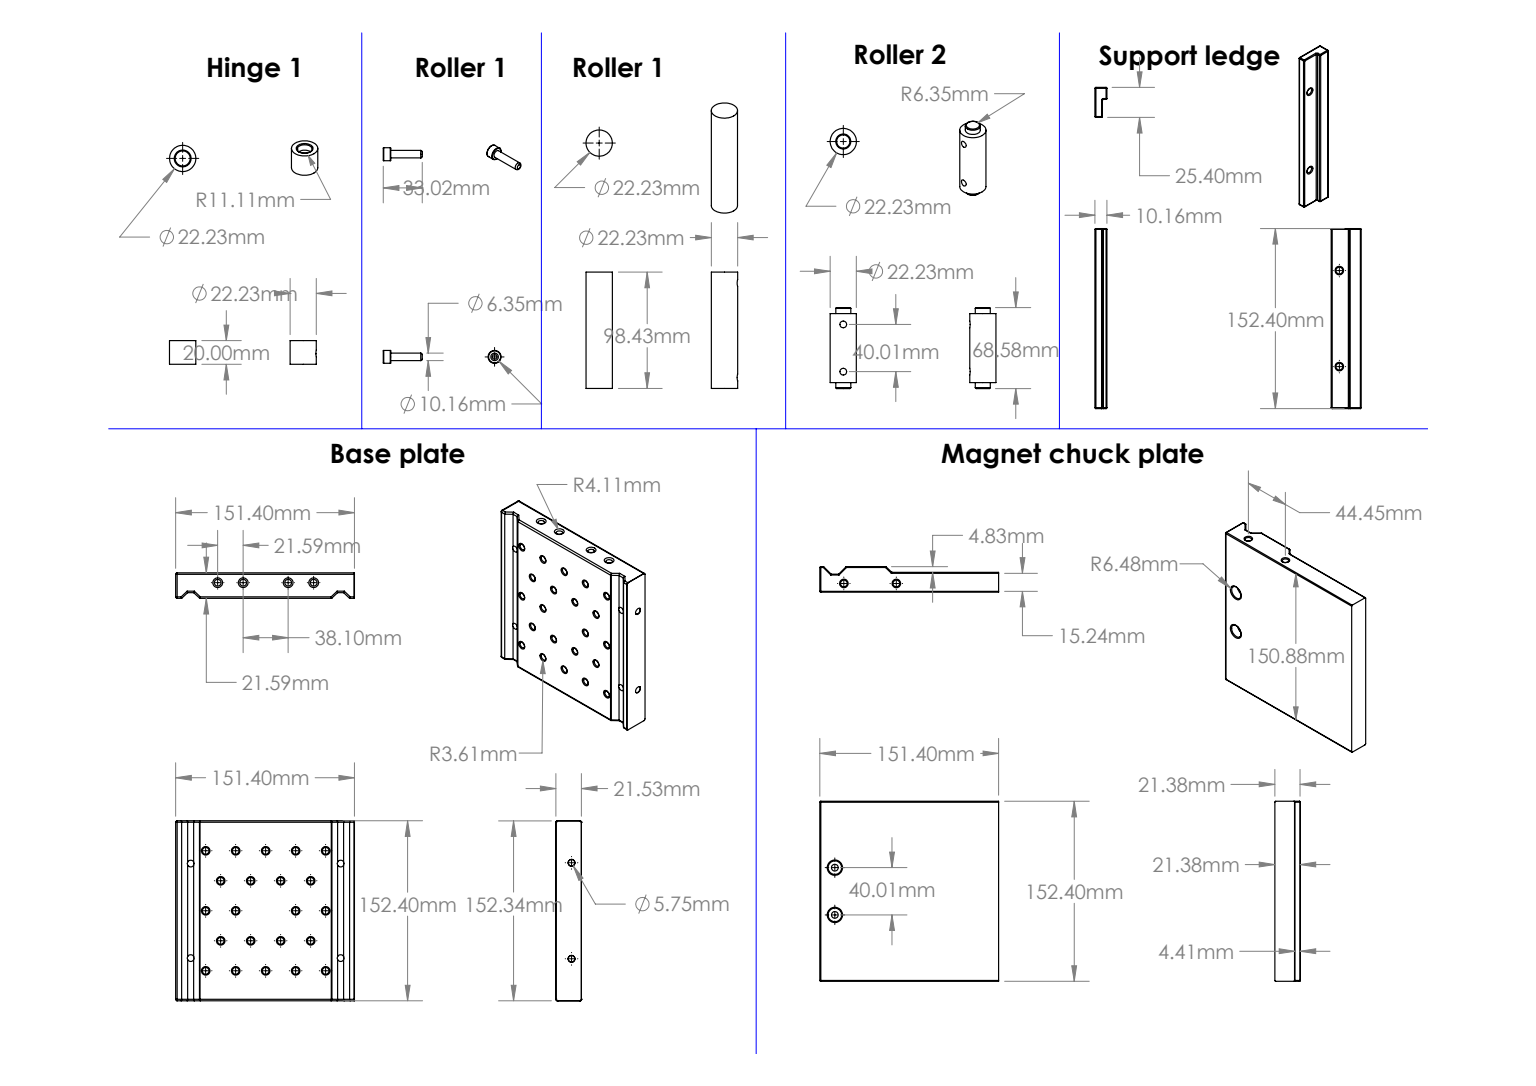
ISO-10303-21;
HEADER;
FILE_DESCRIPTION (('STEP AP214'),
    '1' );
FILE_NAME ('Magnet Chuck Plate.step',
    '2026-10-26T17:37:43',
    ( '' ),
    ( '' ),
    'SwSTEP 2.0',
    'SolidWorks 2024',
    '' );
FILE_SCHEMA (( 'AUTOMOTIVE_DESIGN' ));
ENDSEC;

DATA;
#1=EDGE_CURVE ( 'NONE', #5531, #18286, #22565, .T. ) ;
#10=CARTESIAN_POINT ( 'NONE',  ( 0.7620000000000000107, -3544.061999999999898, 2275.763800000000174 ) ) ;
#53=LINE ( 'NONE', #7432, #17005 ) ;
#82=LINE ( 'NONE', #12499, #17173 ) ;
#90=DIRECTION ( 'NONE',  ( 1.000000000000000000, 0.000000000000000000, 0.000000000000000000 ) ) ;
#100=ORIENTED_EDGE ( 'NONE', *, *, #20293, .T. ) ;
#116=ADVANCED_FACE ( 'NONE', ( #12202 ), #6711, .T. ) ;
#142=DIRECTION ( 'NONE',  ( 0.000000000000000000, 0.000000000000000000, 1.000000000000000000 ) ) ;
#171=DIRECTION ( 'NONE',  ( 0.000000000000000000, 1.000000000000000000, 0.000000000000000000 ) ) ;
#180=AXIS2_PLACEMENT_3D ( 'NONE', #4106, #4219, #18284 ) ;
#191=CARTESIAN_POINT ( 'NONE',  ( 20.32000000000000028, -3568.700000000000273, 2289.213099999999940 ) ) ;
#194=AXIS2_PLACEMENT_3D ( 'NONE', #19267, #12347, #20783 ) ;
#208=CARTESIAN_POINT ( 'NONE',  ( 64.76999999999999602, -3544.061999999999898, 2285.606299999999919 ) ) ;
#211=EDGE_CURVE ( 'NONE', #9937, #6734, #5182, .T. ) ;
#225=ORIENTED_EDGE ( 'NONE', *, *, #4542, .T. ) ;
#244=CIRCLE ( 'NONE', #16685, 5.714999999998999769 ) ;
#250=VECTOR ( 'NONE', #21152, 1000.000000000000000 ) ;
#253=CARTESIAN_POINT ( 'NONE',  ( 64.76999999999999602, -3543.299999999999727, 2289.213099999999940 ) ) ;
#254=ADVANCED_FACE ( 'NONE', ( #12432 ), #16297, .F. ) ;
#255=ADVANCED_FACE ( 'NONE', ( #18168 ), #10909, .F. ) ;
#259=DIRECTION ( 'NONE',  ( 0.000000000000000000, -1.000000000000000000, 0.000000000000000000 ) ) ;
#295=DIRECTION ( 'NONE',  ( -9.561467977825806485E-14, 1.000000000000000000, 0.000000000000000000 ) ) ;
#330=CIRCLE ( 'NONE', #16415, 0.7619999999999294005 ) ;
#355=ADVANCED_FACE ( 'NONE', ( #3996 ), #10792, .T. ) ;
#358=DIRECTION ( 'NONE',  ( 0.000000000000000000, 0.000000000000000000, 1.000000000000000000 ) ) ;
#363=AXIS2_PLACEMENT_3D ( 'NONE', #2504, #11180, #9647 ) ;
#389=AXIS2_PLACEMENT_3D ( 'NONE', #3368, #21197, #5143 ) ;
#392=ORIENTED_EDGE ( 'NONE', *, *, #12214, .T. ) ;
#400=CARTESIAN_POINT ( 'NONE',  ( 19.17699999999999960, -3639.502500000000055, 2295.829799999999977 ) ) ;
#403=DIRECTION ( 'NONE',  ( 1.000000000000000000, 0.000000000000000000, 0.000000000000000000 ) ) ;
#414=CIRCLE ( 'NONE', #13497, 3.606800000000021100 ) ;
#415=LINE ( 'NONE', #12612, #10639 ) ;
#438=VECTOR ( 'NONE', #18888, 1000.000000000000000 ) ;
#440=DIRECTION ( 'NONE',  ( 1.000000000000000000, 0.000000000000000000, 0.000000000000000000 ) ) ;
#441=CARTESIAN_POINT ( 'NONE',  ( 55.57575231171000496, -3544.061999999999898, 2275.763800000000174 ) ) ;
#460=TOROIDAL_SURFACE ( 'NONE', #16565, 6.476999999999000224, 0.7620000000000000107 ) ;
#476=AXIS2_PLACEMENT_3D ( 'NONE', #15163, #22181, #14935 ) ;
#492=CARTESIAN_POINT ( 'NONE',  ( 22.54063073453000143, -3695.699999999999818, 2275.763800000000174 ) ) ;
#504=AXIS2_PLACEMENT_3D ( 'NONE', #7643, #14804, #7882 ) ;
#508=ORIENTED_EDGE ( 'NONE', *, *, #16803, .F. ) ;
#510=CARTESIAN_POINT ( 'NONE',  ( 61.26424768829000556, -3695.699999999999818, 2280.589800000000196 ) ) ;
#520=LINE ( 'NONE', #7549, #8680 ) ;
#522=DIRECTION ( 'NONE',  ( 0.000000000000000000, 0.000000000000000000, 1.000000000000000000 ) ) ;
#555=ORIENTED_EDGE ( 'NONE', *, *, #7128, .T. ) ;
#580=DIRECTION ( 'NONE',  ( 0.000000000000000000, 0.000000000000000000, 1.000000000000000000 ) ) ;
#599=DIRECTION ( 'NONE',  ( 0.000000000000000000, 0.000000000000000000, 1.000000000000000000 ) ) ;
#602=ORIENTED_EDGE ( 'NONE', *, *, #20236, .T. ) ;
#616=ORIENTED_EDGE ( 'NONE', *, *, #16446, .F. ) ;
#626=AXIS2_PLACEMENT_3D ( 'NONE', #6837, #15624, #3186 ) ;
#629=DIRECTION ( 'NONE',  ( -1.000000000000000000, 0.000000000000000000, 0.000000000000000000 ) ) ;
#636=DIRECTION ( 'NONE',  ( 0.000000000000000000, -1.000000000000000000, 0.000000000000000000 ) ) ;
#649=AXIS2_PLACEMENT_3D ( 'NONE', #3890, #6955, #18185 ) ;
#651=ORIENTED_EDGE ( 'NONE', *, *, #14900, .F. ) ;
#654=DIRECTION ( 'NONE',  ( 0.000000000000000000, -1.000000000000000000, 0.000000000000000000 ) ) ;
#661=ADVANCED_FACE ( 'NONE', ( #9884 ), #22307, .T. ) ;
#665=AXIS2_PLACEMENT_3D ( 'NONE', #11297, #7552, #21854 ) ;
#701=ORIENTED_EDGE ( 'NONE', *, *, #13282, .T. ) ;
#725=LINE ( 'NONE', #14924, #438 ) ;
#743=DIRECTION ( 'NONE',  ( 0.000000000000000000, 0.000000000000000000, 1.000000000000000000 ) ) ;
#753=DIRECTION ( 'NONE',  ( -0.7071067811865975328, 0.000000000000000000, 0.7071067811864976127 ) ) ;
#762=EDGE_CURVE ( 'NONE', #1396, #13309, #12722, .T. ) ;
#789=CARTESIAN_POINT ( 'NONE',  ( 22.54063073453000143, -3543.299999999999727, 2275.763800000000174 ) ) ;
#821=DIRECTION ( 'NONE',  ( 0.000000000000000000, 0.000000000000000000, 1.000000000000000000 ) ) ;
#833=VERTEX_POINT ( 'NONE', #22769 ) ;
#834=ORIENTED_EDGE ( 'NONE', *, *, #2199, .T. ) ;
#841=FACE_OUTER_BOUND ( 'NONE', #17125, .T. ) ;
#851=ADVANCED_FACE ( 'NONE', ( #4969 ), #12116, .T. ) ;
#852=AXIS2_PLACEMENT_3D ( 'NONE', #21590, #20065, #5891 ) ;
#864=AXIS2_PLACEMENT_3D ( 'NONE', #15935, #8563, #21219 ) ;
#877=EDGE_LOOP ( 'NONE', ( #14414, #4341, #3151, #7613 ) ) ;
#880=DIRECTION ( 'NONE',  ( 1.000000000000000000, -0.000000000000000000, 1.224646799147353207E-16 ) ) ;
#885=ORIENTED_EDGE ( 'NONE', *, *, #19026, .T. ) ;
#915=DIRECTION ( 'NONE',  ( 1.000000000000000000, 0.000000000000000000, 0.000000000000000000 ) ) ;
#927=VECTOR ( 'NONE', #17929, 1000.000000000000000 ) ;
#942=ADVANCED_FACE ( 'NONE', ( #18087 ), #11055, .F. ) ;
#944=EDGE_CURVE ( 'NONE', #12459, #5100, #7542, .T. ) ;
#948=DIRECTION ( 'NONE',  ( 1.000000000000000000, 0.000000000000000000, 0.000000000000000000 ) ) ;
#993=LINE ( 'NONE', #6058, #8747 ) ;
#1013=DIRECTION ( 'NONE',  ( 0.000000000000000000, 0.000000000000000000, -1.000000000000000000 ) ) ;
#1036=ORIENTED_EDGE ( 'NONE', *, *, #20193, .F. ) ;
#1047=EDGE_LOOP ( 'NONE', ( #19998, #10354 ) ) ;
#1048=AXIS2_PLACEMENT_3D ( 'NONE', #4123, #18073, #7418 ) ;
#1052=EDGE_CURVE ( 'NONE', #8155, #9937, #725, .T. ) ;
#1069=ORIENTED_EDGE ( 'NONE', *, *, #7661, .F. ) ;
#1071=FACE_OUTER_BOUND ( 'NONE', #18282, .T. ) ;
#1081=AXIS2_PLACEMENT_3D ( 'NONE', #4745, #21035, #19158 ) ;
#1088=CARTESIAN_POINT ( 'NONE',  ( 2.859369265564648099, -3695.699999999999818, 2275.763800000091578 ) ) ;
#1109=AXIS2_PLACEMENT_3D ( 'NONE', #7606, #2336, #580 ) ;
#1134=VECTOR ( 'NONE', #15380, 1000.000000000000000 ) ;
#1151=DIRECTION ( 'NONE',  ( -0.6887494619146010688, 0.000000000000000000, 0.7249994335945012525 ) ) ;
#1177=CARTESIAN_POINT ( 'NONE',  ( 12.69999999999999929, -3599.497499999999945, 2288.971800000000258 ) ) ;
#1200=VERTEX_POINT ( 'NONE', #8469 ) ;
#1205=VERTEX_POINT ( 'NONE', #3299 ) ;
#1219=CARTESIAN_POINT ( 'NONE',  ( 64.76999999999999602, -3670.300000000000182, 2286.368300000000090 ) ) ;
#1222=ORIENTED_EDGE ( 'NONE', *, *, #2628, .T. ) ;
#1255=APPLICATION_CONTEXT ( 'configuration controlled 3d designs of mechanical parts and assemblies' ) ;
#1261=ADVANCED_FACE ( 'NONE', ( #17474 ), #5308, .T. ) ;
#1281=DIRECTION ( 'NONE',  ( 0.000000000000000000, 1.000000000000000000, 0.000000000000000000 ) ) ;
#1300=FACE_OUTER_BOUND ( 'NONE', #22874, .T. ) ;
#1301=VECTOR ( 'NONE', #7650, 1000.000000000000000 ) ;
#1306=DIRECTION ( 'NONE',  ( 0.000000000000000000, 0.000000000000000000, 1.000000000000000000 ) ) ;
#1321=CARTESIAN_POINT ( 'NONE',  ( 22.00181536726000076, -3694.938000000000102, 2275.224984633000076 ) ) ;
#1325=ADVANCED_FACE ( 'NONE', ( #21119 ), #14206, .F. ) ;
#1327=ORIENTED_EDGE ( 'NONE', *, *, #3052, .T. ) ;
#1343=EDGE_LOOP ( 'NONE', ( #9952, #15116, #508, #11219 ) ) ;
#1358=VECTOR ( 'NONE', #19375, 1000.000000000000000 ) ;
#1371=VERTEX_POINT ( 'NONE', #21695 ) ;
#1372=CIRCLE ( 'NONE', #12234, 5.714999999999999858 ) ;
#1396=VERTEX_POINT ( 'NONE', #17830 ) ;
#1409=CARTESIAN_POINT ( 'NONE',  ( 12.69999999999999929, -3599.497499999999945, 2296.591799999999694 ) ) ;
#1411=AXIS2_PLACEMENT_3D ( 'NONE', #10840, #17987, #14487 ) ;
#1414=VERTEX_POINT ( 'NONE', #7284 ) ;
#1421=SHAPE_REPRESENTATION ( 'Magnet Chuck Plate', ( #5611 ), #15735 ) ;
#1423=DIRECTION ( 'NONE',  ( 1.000000000000000000, 0.000000000000000000, 0.000000000000000000 ) ) ;
#1426=CARTESIAN_POINT ( 'NONE',  ( 61.26424768829000556, -3544.061999999999898, 2279.065800000000309 ) ) ;
#1428=DIRECTION ( 'NONE',  ( 0.000000000000000000, 0.000000000000000000, 1.000000000000000000 ) ) ;
#1439=CIRCLE ( 'NONE', #4438, 0.7619999999999294005 ) ;
#1444=CARTESIAN_POINT ( 'NONE',  ( 55.57575231171000496, -3544.061999999999898, 2275.001800000000003 ) ) ;
#1482=CARTESIAN_POINT ( 'NONE',  ( 6.985000000000999520, -3599.497499999999945, 2288.971800000000258 ) ) ;
#1484=VERTEX_POINT ( 'NONE', #13128 ) ;
#1496=ORIENTED_EDGE ( 'NONE', *, *, #16738, .F. ) ;
#1502=CARTESIAN_POINT ( 'NONE',  ( 20.32000000000000028, -3670.300000000000182, 2286.368300000000090 ) ) ;
#1509=EDGE_CURVE ( 'NONE', #7148, #4633, #7924, .T. ) ;
#1513=DIRECTION ( 'NONE',  ( 0.000000000000000000, 0.000000000000000000, 1.000000000000000000 ) ) ;
#1519=DIRECTION ( 'NONE',  ( -0.7071067811860285435, 0.000000000000000000, -0.7071067811870666020 ) ) ;
#1533=ORIENTED_EDGE ( 'NONE', *, *, #7543, .T. ) ;
#1537=ORIENTED_EDGE ( 'NONE', *, *, #16396, .F. ) ;
#1551=CARTESIAN_POINT ( 'NONE',  ( 151.6380000000000052, -3544.061999999999898, 2279.827800000000025 ) ) ;
#1558=EDGE_LOOP ( 'NONE', ( #1774, #9639 ) ) ;
#1571=ORIENTED_EDGE ( 'NONE', *, *, #2628, .F. ) ;
#1574=CARTESIAN_POINT ( 'NONE',  ( 11.65131536725999872, -3544.061999999999898, 2286.653115367000282 ) ) ;
#1584=DIRECTION ( 'NONE',  ( 0.000000000000000000, 1.000000000000000000, 0.000000000000000000 ) ) ;
#1589=CARTESIAN_POINT ( 'NONE',  ( 152.4000000000000057, -3694.938000000000102, 2295.829799999999977 ) ) ;
#1609=VECTOR ( 'NONE', #2505, 1000.000000000000000 ) ;
#1614=ORIENTED_EDGE ( 'NONE', *, *, #9995, .F. ) ;
#1626=ORIENTED_EDGE ( 'NONE', *, *, #3283, .F. ) ;
#1631=ORIENTED_EDGE ( 'NONE', *, *, #8221, .F. ) ;
#1632=CARTESIAN_POINT ( 'NONE',  ( 9.209369265603214672, -3695.699999999999818, 2282.113800000000083 ) ) ;
#1653=CIRCLE ( 'NONE', #15143, 2.844800000000091700 ) ;
#1658=FACE_OUTER_BOUND ( 'NONE', #3586, .T. ) ;
#1687=EDGE_LOOP ( 'NONE', ( #8535, #1801, #12779, #20172 ) ) ;
#1690=CARTESIAN_POINT ( 'NONE',  ( 20.32000000000000028, -3568.700000000000273, 2289.213099999999940 ) ) ;
#1696=AXIS2_PLACEMENT_3D ( 'NONE', #22716, #22825, #10413 ) ;
#1702=CARTESIAN_POINT ( 'NONE',  ( 55.57575231171000496, -3544.061999999999898, 2275.001800000000003 ) ) ;
#1703=DIRECTION ( 'NONE',  ( 0.000000000000000000, 0.000000000000000000, -1.000000000000000000 ) ) ;
#1724=CARTESIAN_POINT ( 'NONE',  ( 55.57575231171000496, -3695.699999999999818, 2275.763800000000174 ) ) ;
#1729=DIRECTION ( 'NONE',  ( 0.000000000000000000, 0.000000000000000000, -1.000000000000000000 ) ) ;
#1734=DIRECTION ( 'NONE',  ( 0.000000000000000000, -1.000000000000000000, 0.000000000000000000 ) ) ;
#1736=LINE ( 'NONE', #5020, #1956 ) ;
#1742=VERTEX_POINT ( 'NONE', #2106 ) ;
#1743=DIRECTION ( 'NONE',  ( 0.000000000000000000, 0.000000000000000000, 1.000000000000000000 ) ) ;
#1770=CARTESIAN_POINT ( 'NONE',  ( 64.76999999999999602, -3544.061999999999898, 2289.213099999999940 ) ) ;
#1774=ORIENTED_EDGE ( 'NONE', *, *, #4675, .T. ) ;
#1778=EDGE_LOOP ( 'NONE', ( #14987, #13379, #9900, #1833 ) ) ;
#1783=LINE ( 'NONE', #8929, #16569 ) ;
#1794=CYLINDRICAL_SURFACE ( 'NONE', #11682, 0.7620000000000000107 ) ;
#1795=EDGE_CURVE ( 'NONE', #1396, #6791, #16164, .T. ) ;
#1801=ORIENTED_EDGE ( 'NONE', *, *, #7994, .T. ) ;
#1814=CARTESIAN_POINT ( 'NONE',  ( 151.4000000000000057, -3543.299999999999727, 2279.827800000000025 ) ) ;
#1819=DIRECTION ( 'NONE',  ( 0.000000000000000000, 0.000000000000000000, -1.000000000000000000 ) ) ;
#1832=DIRECTION ( 'NONE',  ( 0.000000000000000000, 0.000000000000000000, 1.000000000000000000 ) ) ;
#1833=ORIENTED_EDGE ( 'NONE', *, *, #10605, .F. ) ;
#1845=DIRECTION ( 'NONE',  ( 0.000000000000000000, 0.000000000000000000, 1.000000000000000000 ) ) ;
#1847=EDGE_CURVE ( 'NONE', #21628, #1200, #1864, .T. ) ;
#1859=DIRECTION ( 'NONE',  ( 0.000000000000000000, 0.000000000000000000, -1.000000000000000000 ) ) ;
#1862=ORIENTED_EDGE ( 'NONE', *, *, #23159, .F. ) ;
#1864=LINE ( 'NONE', #11124, #7577 ) ;
#1888=FACE_OUTER_BOUND ( 'NONE', #14803, .T. ) ;
#1901=CARTESIAN_POINT ( 'NONE',  ( 151.4000000000000057, 0.000000000000000000, 0.000000000000000000 ) ) ;
#1918=DIRECTION ( 'NONE',  ( 0.000000000000000000, 0.000000000000000000, 1.000000000000000000 ) ) ;
#1927=FACE_BOUND ( 'NONE', #9861, .T. ) ;
#1930=CARTESIAN_POINT ( 'NONE',  ( 12.69999999999999929, -3639.502500000000055, 2288.971800000000258 ) ) ;
#1933=EDGE_LOOP ( 'NONE', ( #7935, #18897, #1571, #14077 ) ) ;
#1940=CARTESIAN_POINT ( 'NONE',  ( 151.4000000000000057, -3544.061999999999898, 2295.829799999999977 ) ) ;
#1956=VECTOR ( 'NONE', #8650, 1000.000000000000000 ) ;
#1972=VECTOR ( 'NONE', #3362, 1000.000000000000000 ) ;
#1978=AXIS2_PLACEMENT_3D ( 'NONE', #20945, #19307, #6893 ) ;
#2003=CARTESIAN_POINT ( 'NONE',  ( 6.985000000000999520, -3599.497499999999945, 2288.971800000000258 ) ) ;
#2010=AXIS2_PLACEMENT_3D ( 'NONE', #12669, #259, #11022 ) ;
#2012=DIRECTION ( 'NONE',  ( 1.000000000000000000, 0.000000000000000000, 0.000000000000000000 ) ) ;
#2028=VERTEX_POINT ( 'NONE', #16615 ) ;
#2034=VECTOR ( 'NONE', #13795, 1000.000000000000000 ) ;
#2045=DIRECTION ( 'NONE',  ( -1.000000000000000000, 0.000000000000000000, 0.000000000000000000 ) ) ;
#2058=VERTEX_POINT ( 'NONE', #4314 ) ;
#2098=EDGE_CURVE ( 'NONE', #833, #9227, #19190, .T. ) ;
#2106=CARTESIAN_POINT ( 'NONE',  ( 64.76999999999999602, -3695.699999999999818, 2292.819899999999961 ) ) ;
#2128=EDGE_CURVE ( 'NONE', #19405, #9540, #6099, .T. ) ;
#2134=ORIENTED_EDGE ( 'NONE', *, *, #9935, .F. ) ;
#2147=FACE_OUTER_BOUND ( 'NONE', #19239, .T. ) ;
#2152=VECTOR ( 'NONE', #4453, 1000.000000000000000 ) ;
#2162=DIRECTION ( 'NONE',  ( -1.000000000000000000, 0.000000000000000000, 0.000000000000000000 ) ) ;
#2169=LINE ( 'NONE', #15042, #9720 ) ;
#2170=CARTESIAN_POINT ( 'NONE',  ( 22.54063073453000143, -3544.061999999999898, 2275.763800000000174 ) ) ;
#2175=CARTESIAN_POINT ( 'NONE',  ( 12.69999999999999929, -3599.497499999999945, 2295.829799999999977 ) ) ;
#2199=EDGE_CURVE ( 'NONE', #17590, #16242, #20830, .T. ) ;
#2200=DIRECTION ( 'NONE',  ( 0.000000000000000000, 1.000000000000000000, 0.000000000000000000 ) ) ;
#2202=ADVANCED_FACE ( 'NONE', ( #11920 ), #19067, .F. ) ;
#2207=FACE_OUTER_BOUND ( 'NONE', #7045, .T. ) ;
#2257=( GEOMETRIC_REPRESENTATION_CONTEXT ( 3 ) GLOBAL_UNCERTAINTY_ASSIGNED_CONTEXT ( ( #16741 ) ) GLOBAL_UNIT_ASSIGNED_CONTEXT ( ( #21126, #3419, #23094 ) ) REPRESENTATION_CONTEXT ( 'NONE', 'WORKASPACE' ) );
#2264=ORIENTED_EDGE ( 'NONE', *, *, #19899, .F. ) ;
#2279=DIRECTION ( 'NONE',  ( -1.000000000000000000, 0.000000000000000000, 0.000000000000000000 ) ) ;
#2294=AXIS2_PLACEMENT_3D ( 'NONE', #19270, #3205, #8606 ) ;
#2301=LINE ( 'NONE', #6164, #9335 ) ;
#2320=FACE_OUTER_BOUND ( 'NONE', #12713, .T. ) ;
#2336=DIRECTION ( 'NONE',  ( 0.000000000000000000, 1.000000000000000000, 0.000000000000000000 ) ) ;
#2367=CARTESIAN_POINT ( 'NONE',  ( 19.17699999999900129, -3599.497499999999945, 2296.591799999999694 ) ) ;
#2377=ORIENTED_EDGE ( 'NONE', *, *, #14900, .T. ) ;
#2403=ORIENTED_EDGE ( 'NONE', *, *, #12414, .T. ) ;
#2416=EDGE_CURVE ( 'NONE', #18510, #16618, #10097, .T. ) ;
#2424=EDGE_CURVE ( 'NONE', #5311, #11834, #20766, .T. ) ;
#2442=ORIENTED_EDGE ( 'NONE', *, *, #4508, .T. ) ;
#2445=VERTEX_POINT ( 'NONE', #5946 ) ;
#2446=VERTEX_POINT ( 'NONE', #23092 ) ;
#2449=AXIS2_PLACEMENT_3D ( 'NONE', #1177, #6824, #17472 ) ;
#2491=AXIS2_PLACEMENT_3D ( 'NONE', #5799, #7435, #14474 ) ;
#2502=VECTOR ( 'NONE', #7547, 1000.000000000000000 ) ;
#2504=CARTESIAN_POINT ( 'NONE',  ( 151.4000000000000057, -3544.061999999999898, 2280.589800000000196 ) ) ;
#2505=DIRECTION ( 'NONE',  ( 0.7249994335945980639, 0.000000000000000000, 0.6887494619144990393 ) ) ;
#2509=CYLINDRICAL_SURFACE ( 'NONE', #12038, 0.7619999999999294005 ) ;
#2511=ADVANCED_FACE ( 'NONE', ( #19247 ), #12830, .T. ) ;
#2515=AXIS2_PLACEMENT_3D ( 'NONE', #16875, #9960, #821 ) ;
#2521=ORIENTED_EDGE ( 'NONE', *, *, #944, .F. ) ;
#2522=ORIENTED_EDGE ( 'NONE', *, *, #9271, .T. ) ;
#2526=DIRECTION ( 'NONE',  ( 1.122008997397786234E-13, 0.000000000000000000, 1.000000000000000000 ) ) ;
#2534=CIRCLE ( 'NONE', #22730, 0.7619999999999294005 ) ;
#2536=VECTOR ( 'NONE', #522, 1000.000000000000000 ) ;
#2537=CARTESIAN_POINT ( 'NONE',  ( 0.000000000000000000, -3543.299999999999727, 2275.001800000000003 ) ) ;
#2541=EDGE_CURVE ( 'NONE', #5311, #1396, #22914, .T. ) ;
#2579=EDGE_CURVE ( 'NONE', #12459, #7148, #1783, .T. ) ;
#2598=ORIENTED_EDGE ( 'NONE', *, *, #22441, .T. ) ;
#2602=LINE ( 'NONE', #16558, #1301 ) ;
#2606=CARTESIAN_POINT ( 'NONE',  ( 0.000000000000000000, 0.000000000000000000, 0.000000000000000000 ) ) ;
#2609=CIRCLE ( 'NONE', #6035, 2.844799999999999773 ) ;
#2628=EDGE_CURVE ( 'NONE', #12083, #15238, #6115, .T. ) ;
#2649=DIRECTION ( 'NONE',  ( 0.000000000000000000, 0.000000000000000000, 1.000000000000000000 ) ) ;
#2654=DIRECTION ( 'NONE',  ( 0.000000000000000000, 1.000000000000000000, 0.000000000000000000 ) ) ;
#2694=AXIS2_PLACEMENT_3D ( 'NONE', #9503, #19719, #17943 ) ;
#2695=ORIENTED_EDGE ( 'NONE', *, *, #1052, .F. ) ;
#2697=DIRECTION ( 'NONE',  ( 1.000000000000000000, 0.000000000000000000, 0.000000000000000000 ) ) ;
#2711=DIRECTION ( 'NONE',  ( -0.000000000000000000, -1.000000000000000000, -0.000000000000000000 ) ) ;
#2732=ORIENTED_EDGE ( 'NONE', *, *, #211, .T. ) ;
#2759=DIRECTION ( 'NONE',  ( 0.000000000000000000, 0.000000000000000000, 1.000000000000000000 ) ) ;
#2761=FACE_OUTER_BOUND ( 'NONE', #22142, .T. ) ;
#2776=EDGE_CURVE ( 'NONE', #19948, #2028, #13473, .T. ) ;
#2797=DIRECTION ( 'NONE',  ( 0.000000000000000000, 1.000000000000000000, 0.000000000000000000 ) ) ;
#2799=ORIENTED_EDGE ( 'NONE', *, *, #18836, .F. ) ;
#2806=VERTEX_POINT ( 'NONE', #13363 ) ;
#2807=AXIS2_PLACEMENT_3D ( 'NONE', #17091, #1151, #2797 ) ;
#2809=DIRECTION ( 'NONE',  ( 0.000000000000000000, 0.000000000000000000, 1.000000000000000000 ) ) ;
#2824=EDGE_CURVE ( 'NONE', #16618, #7940, #22254, .T. ) ;
#2831=VECTOR ( 'NONE', #15386, 1000.000000000000000 ) ;
#2854=ORIENTED_EDGE ( 'NONE', *, *, #23159, .T. ) ;
#2890=DIRECTION ( 'NONE',  ( 0.000000000000000000, -1.000000000000000000, 0.000000000000000000 ) ) ;
#2904=SPHERICAL_SURFACE ( 'NONE', #6798, 0.7620000000000000107 ) ;
#2913=VECTOR ( 'NONE', #11235, 1000.000000000000000 ) ;
#2924=EDGE_CURVE ( 'NONE', #9308, #12115, #4684, .T. ) ;
#2925=ORIENTED_EDGE ( 'NONE', *, *, #9144, .T. ) ;
#2929=EDGE_CURVE ( 'NONE', #19560, #20662, #244, .T. ) ;
#2931=DIRECTION ( 'NONE',  ( -0.7071067811865969777, 0.000000000000000000, 0.7071067811864980568 ) ) ;
#2950=DIRECTION ( 'NONE',  ( -0.000000000000000000, 1.000000000000000000, 0.000000000000000000 ) ) ;
#2956=LINE ( 'NONE', #10102, #11863 ) ;
#2962=CARTESIAN_POINT ( 'NONE',  ( 64.76999999999999602, -3543.299999999999727, 2292.819899999999961 ) ) ;
#2971=CARTESIAN_POINT ( 'NONE',  ( 22.54063073453000143, -3543.299999999999727, 2275.763800000000174 ) ) ;
#2985=EDGE_LOOP ( 'NONE', ( #23150, #7018, #9034, #15531 ) ) ;
#3000=EDGE_CURVE ( 'NONE', #7148, #2806, #18196, .T. ) ;
#3019=DIRECTION ( 'NONE',  ( -1.000000000000000000, 0.000000000000000000, 0.000000000000000000 ) ) ;
#3039=DIRECTION ( 'NONE',  ( 0.000000000000000000, 0.000000000000000000, -1.000000000000000000 ) ) ;
#3043=FACE_OUTER_BOUND ( 'NONE', #6602, .T. ) ;
#3048=AXIS2_PLACEMENT_3D ( 'NONE', #21363, #17950, #10923 ) ;
#3052=EDGE_CURVE ( 'NONE', #3812, #9191, #6694, .T. ) ;
#3066=VECTOR ( 'NONE', #16390, 1000.000000000000000 ) ;
#3071=DIRECTION ( 'NONE',  ( 0.7071067811865975328, -3.219513736388853369E-15, -0.7071067811864976127 ) ) ;
#3077=AXIS2_PLACEMENT_3D ( 'NONE', #2537, #15190, #20350 ) ;
#3085=ORIENTED_EDGE ( 'NONE', *, *, #762, .F. ) ;
#3086=CARTESIAN_POINT ( 'NONE',  ( 3.044261469286652755, -3695.700000000080308, 2275.317430734601658 ) ) ;
#3107=FACE_OUTER_BOUND ( 'NONE', #14452, .T. ) ;
#3109=AXIS2_PLACEMENT_3D ( 'NONE', #10, #9029, #5176 ) ;
#3120=ADVANCED_FACE ( 'NONE', ( #6916, #13946, #21095 ), #12184, .F. ) ;
#3151=ORIENTED_EDGE ( 'NONE', *, *, #22542, .T. ) ;
#3166=ORIENTED_EDGE ( 'NONE', *, *, #9981, .T. ) ;
#3181=DIRECTION ( 'NONE',  ( -1.000000000000000000, 0.000000000000000000, 0.000000000000000000 ) ) ;
#3186=DIRECTION ( 'NONE',  ( 1.000000000000000000, 0.000000000000000000, 0.000000000000000000 ) ) ;
#3192=VECTOR ( 'NONE', #8691, 1000.000000000000000 ) ;
#3205=DIRECTION ( 'NONE',  ( -0.7071067811865975328, 0.000000000000000000, -0.7071067811864976127 ) ) ;
#3213=FACE_OUTER_BOUND ( 'NONE', #14947, .T. ) ;
#3230=VERTEX_POINT ( 'NONE', #20574 ) ;
#3232=AXIS2_PLACEMENT_3D ( 'NONE', #8008, #16897, #22056 ) ;
#3233=CARTESIAN_POINT ( 'NONE',  ( 20.32000000000000028, -3694.938000000000102, 2289.213099999999940 ) ) ;
#3237=DIRECTION ( 'NONE',  ( 0.000000000000000000, -1.000000000000000000, 0.000000000000000000 ) ) ;
#3238=LINE ( 'NONE', #8401, #4699 ) ;
#3275=CARTESIAN_POINT ( 'NONE',  ( 15.87500000000000000, -3543.299999999999727, 2281.351799999999912 ) ) ;
#3277=AXIS2_PLACEMENT_3D ( 'NONE', #18323, #2045, #9314 ) ;
#3283=EDGE_CURVE ( 'NONE', #9572, #19328, #7733, .T. ) ;
#3297=ORIENTED_EDGE ( 'NONE', *, *, #18597, .T. ) ;
#3299=CARTESIAN_POINT ( 'NONE',  ( 15.54479999999999862, -3599.497499999999945, 2281.351799999999912 ) ) ;
#3307=DIRECTION ( 'NONE',  ( 2.294752314678193758E-12, 0.000000000000000000, 1.000000000000000000 ) ) ;
#3308=FACE_OUTER_BOUND ( 'NONE', #15006, .T. ) ;
#3311=EDGE_LOOP ( 'NONE', ( #5703, #20308, #885, #21896 ) ) ;
#3313=DIRECTION ( 'NONE',  ( 1.000000000000000000, 0.000000000000000000, 0.000000000000000000 ) ) ;
#3339=ORIENTED_EDGE ( 'NONE', *, *, #14329, .F. ) ;
#3350=APPLICATION_CONTEXT ( 'configuration controlled 3d designs of mechanical parts and assemblies' ) ;
#3362=DIRECTION ( 'NONE',  ( 0.000000000000000000, 0.000000000000000000, 1.000000000000000000 ) ) ;
#3368=CARTESIAN_POINT ( 'NONE',  ( 20.32000000000000028, -3694.938000000000102, 2292.819899999999961 ) ) ;
#3387=ORIENTED_EDGE ( 'NONE', *, *, #9144, .F. ) ;
#3403=ORIENTED_EDGE ( 'NONE', *, *, #5149, .T. ) ;
#3405=AXIS2_PLACEMENT_3D ( 'NONE', #20547, #13294, #18573 ) ;
#3410=ADVANCED_FACE ( 'NONE', ( #21054 ), #14257, .T. ) ;
#3415=DIRECTION ( 'NONE',  ( 0.000000000000000000, -1.000000000000000000, 0.000000000000000000 ) ) ;
#3419=( NAMED_UNIT ( * ) PLANE_ANGLE_UNIT ( ) SI_UNIT ( $, .RADIAN. ) );
#3427=CARTESIAN_POINT ( 'NONE',  ( 20.32000000000000028, -3544.061999999999898, 2286.368300000000090 ) ) ;
#3430=EDGE_CURVE ( 'NONE', #2806, #6290, #11126, .T. ) ;
#3435=EDGE_LOOP ( 'NONE', ( #15644, #22881, #10435, #22509 ) ) ;
#3437=AXIS2_PLACEMENT_3D ( 'NONE', #9950, #18739, #5888 ) ;
#3454=CIRCLE ( 'NONE', #2694, 2.844800000000091700 ) ;
#3525=AXIS2_PLACEMENT_3D ( 'NONE', #18593, #9791, #11657 ) ;
#3534=ORIENTED_EDGE ( 'NONE', *, *, #9315, .F. ) ;
#3539=ADVANCED_FACE ( 'NONE', ( #9095 ), #7560, .F. ) ;
#3548=AXIS2_PLACEMENT_3D ( 'NONE', #7777, #13494, #15149 ) ;
#3563=FACE_BOUND ( 'NONE', #14863, .T. ) ;
#3569=VECTOR ( 'NONE', #2654, 1000.000000000000000 ) ;
#3586=EDGE_LOOP ( 'NONE', ( #10181, #18085, #6846, #6850 ) ) ;
#3623=ORIENTED_EDGE ( 'NONE', *, *, #15602, .T. ) ;
#3632=CARTESIAN_POINT ( 'NONE',  ( 64.76999999999999602, -3694.938000000000102, 2289.213099999999940 ) ) ;
#3638=CARTESIAN_POINT ( 'NONE',  ( 61.26424768829000556, -3544.061999999999898, 2279.827800000000025 ) ) ;
#3647=CYLINDRICAL_SURFACE ( 'NONE', #8054, 2.844800000000091700 ) ;
#3648=ORIENTED_EDGE ( 'NONE', *, *, #2579, .F. ) ;
#3658=ORIENTED_EDGE ( 'NONE', *, *, #9433, .F. ) ;
#3659=CARTESIAN_POINT ( 'NONE',  ( 12.69999999999999929, -3639.502500000000055, 2288.971800000000258 ) ) ;
#3675=CARTESIAN_POINT ( 'NONE',  ( 0.7620000000000000107, -3694.938000000000102, 2296.591799999999694 ) ) ;
#3689=CARTESIAN_POINT ( 'NONE',  ( 151.4000000000000057, -3694.938000000000102, 2279.827800000000025 ) ) ;
#3709=DIRECTION ( 'NONE',  ( 1.122008997397786234E-13, 0.000000000000000000, 1.000000000000000000 ) ) ;
#3716=ADVANCED_FACE ( 'NONE', ( #12334 ), #5553, .T. ) ;
#3721=DIRECTION ( 'NONE',  ( 1.000000000000000000, 0.000000000000000000, 0.000000000000000000 ) ) ;
#3739=LINE ( 'NONE', #3863, #18974 ) ;
#3741=CARTESIAN_POINT ( 'NONE',  ( 61.26424768829000556, -3694.938000000000102, 2279.827800000000025 ) ) ;
#3744=ORIENTED_EDGE ( 'NONE', *, *, #3430, .F. ) ;
#3749=CARTESIAN_POINT ( 'NONE',  ( 0.000000000000000000, -3694.938000000000102, 2275.763800000000174 ) ) ;
#3755=EDGE_LOOP ( 'NONE', ( #10231, #17493, #6970, #18639 ) ) ;
#3779=VERTEX_POINT ( 'NONE', #492 ) ;
#3788=ORIENTED_EDGE ( 'NONE', *, *, #18377, .T. ) ;
#3812=VERTEX_POINT ( 'NONE', #9292 ) ;
#3834=DIRECTION ( 'NONE',  ( -4.553079989440860501E-14, 1.000000000000000000, 0.000000000000000000 ) ) ;
#3848=CIRCLE ( 'NONE', #19952, 2.844800000000091700 ) ;
#3863=CARTESIAN_POINT ( 'NONE',  ( 9.855199999999999960, -3599.497499999999945, 2263.571799999999712 ) ) ;
#3868=AXIS2_PLACEMENT_3D ( 'NONE', #18970, #9820, #13697 ) ;
#3872=CARTESIAN_POINT ( 'NONE',  ( 2.859369265473000077, -3695.699999999999818, 2275.763800000000174 ) ) ;
#3874=CYLINDRICAL_SURFACE ( 'NONE', #17366, 0.7619999999999294005 ) ;
#3890=CARTESIAN_POINT ( 'NONE',  ( 0.000000000000000000, -3544.061999999999898, 2282.113800000000083 ) ) ;
#3895=EDGE_LOOP ( 'NONE', ( #11821, #11206, #16120 ) ) ;
#3900=VERTEX_POINT ( 'NONE', #6004 ) ;
#3901=EDGE_LOOP ( 'NONE', ( #9269, #18319, #22768, #18792 ) ) ;
#3915=FACE_OUTER_BOUND ( 'NONE', #13642, .T. ) ;
#3922=CIRCLE ( 'NONE', #22623, 0.7619999999999294005 ) ;
#3933=AXIS2_PLACEMENT_3D ( 'NONE', #19711, #17934, #17827 ) ;
#3946=EDGE_LOOP ( 'NONE', ( #15587, #17728 ) ) ;
#3954=AXIS2_PLACEMENT_3D ( 'NONE', #10766, #17909, #1859 ) ;
#3957=CARTESIAN_POINT ( 'NONE',  ( 61.26424768829000556, -3543.299999999999727, 2279.065800000000309 ) ) ;
#3959=( BOUNDED_CURVE ( )  B_SPLINE_CURVE ( 3, ( #16933, #11777, #13543, #8392 ),
 .UNSPECIFIED., .F., .T. ) 
 B_SPLINE_CURVE_WITH_KNOTS ( ( 4, 4 ),
 ( 1.570796326732663450, 3.141592653589793116 ),
 .UNSPECIFIED. ) 
 CURVE ( )  GEOMETRIC_REPRESENTATION_ITEM ( )  RATIONAL_B_SPLINE_CURVE ( ( 1.000000000000000000, 0.8047378541096965598, 0.8047378541096965598, 1.000000000000000000 ) ) 
 REPRESENTATION_ITEM ( '' )  );
#3960=CARTESIAN_POINT ( 'NONE',  ( 12.69999999999999929, -3599.497499999999945, 2288.971800000000258 ) ) ;
#3970=ORIENTED_EDGE ( 'NONE', *, *, #15959, .F. ) ;
#3978=VECTOR ( 'NONE', #2931, 1000.000000000000000 ) ;
#3981=EDGE_CURVE ( 'NONE', #10237, #21628, #22378, .T. ) ;
#3996=FACE_OUTER_BOUND ( 'NONE', #1343, .T. ) ;
#4000=DIRECTION ( 'NONE',  ( 0.000000000000000000, 1.000000000000000000, 0.000000000000000000 ) ) ;
#4010=SHAPE_DEFINITION_REPRESENTATION ( #15743, #1421 ) ;
#4017=VERTEX_POINT ( 'NONE', #18751 ) ;
#4027=DIRECTION ( 'NONE',  ( 1.000000000000000000, 0.000000000000000000, 0.000000000000000000 ) ) ;
#4036=DIRECTION ( 'NONE',  ( -1.000000000000000000, 0.000000000000000000, 0.000000000000000000 ) ) ;
#4048=CARTESIAN_POINT ( 'NONE',  ( 16.19063073443439293, -3695.699999999999818, 2282.113800000095125 ) ) ;
#4056=DIRECTION ( 'NONE',  ( 0.000000000000000000, 0.000000000000000000, -1.000000000000000000 ) ) ;
#4097=CARTESIAN_POINT ( 'NONE',  ( 0.7620000000000000107, -3694.938000000000102, 2275.763800000000174 ) ) ;
#4101=EDGE_CURVE ( 'NONE', #6730, #22793, #6003, .T. ) ;
#4104=VERTEX_POINT ( 'NONE', #19806 ) ;
#4106=CARTESIAN_POINT ( 'NONE',  ( 64.76999999999999602, -3544.061999999999898, 2289.213099999999940 ) ) ;
#4123=CARTESIAN_POINT ( 'NONE',  ( 20.32000000000000028, -3695.699999999999818, 2289.213099999999940 ) ) ;
#4167=DIRECTION ( 'NONE',  ( -1.000000000000000000, 0.000000000000000000, 0.000000000000000000 ) ) ;
#4179=CARTESIAN_POINT ( 'NONE',  ( 12.69999999999999929, -3599.497499999999945, 2281.351799999999912 ) ) ;
#4215=ORIENTED_EDGE ( 'NONE', *, *, #4834, .T. ) ;
#4219=DIRECTION ( 'NONE',  ( 0.000000000000000000, -1.000000000000000000, 0.000000000000000000 ) ) ;
#4248=ORIENTED_EDGE ( 'NONE', *, *, #7834, .T. ) ;
#4265=FACE_OUTER_BOUND ( 'NONE', #6709, .T. ) ;
#4286=FACE_OUTER_BOUND ( 'NONE', #12773, .T. ) ;
#4289=DIRECTION ( 'NONE',  ( 0.000000000000000000, 0.000000000000000000, 1.000000000000000000 ) ) ;
#4309=AXIS2_PLACEMENT_3D ( 'NONE', #18288, #4000, #9498 ) ;
#4310=ORIENTED_EDGE ( 'NONE', *, *, #1052, .T. ) ;
#4314=CARTESIAN_POINT ( 'NONE',  ( 60.73942059830999796, -3694.938000000000102, 2279.618249568000010 ) ) ;
#4316=ORIENTED_EDGE ( 'NONE', *, *, #17727, .F. ) ;
#4328=DIRECTION ( 'NONE',  ( 0.000000000000000000, -1.000000000000000000, 0.000000000000000000 ) ) ;
#4329=ADVANCED_FACE ( 'NONE', ( #13222 ), #14600, .T. ) ;
#4341=ORIENTED_EDGE ( 'NONE', *, *, #11287, .F. ) ;
#4349=ORIENTED_EDGE ( 'NONE', *, *, #944, .T. ) ;
#4358=CIRCLE ( 'NONE', #19331, 6.477000000000000313 ) ;
#4399=CARTESIAN_POINT ( 'NONE',  ( 9.524999999998000177, -3543.299999999999727, 2281.351799999999912 ) ) ;
#4400=CARTESIAN_POINT ( 'NONE',  ( 22.76381536726000121, -3694.938000000000102, 2275.540615367000555 ) ) ;
#4403=CARTESIAN_POINT ( 'NONE',  ( 2.859369265602505816, -3543.299999999999727, 2275.763800000000629 ) ) ;
#4409=VECTOR ( 'NONE', #20650, 1000.000000000000000 ) ;
#4413=LINE ( 'NONE', #17395, #12601 ) ;
#4417=DIRECTION ( 'NONE',  ( 0.000000000000000000, 0.000000000000000000, 1.000000000000000000 ) ) ;
#4421=CARTESIAN_POINT ( 'NONE',  ( 20.32000000000000028, -3544.061999999999898, 2289.213099999999940 ) ) ;
#4431=ORIENTED_EDGE ( 'NONE', *, *, #10605, .T. ) ;
#4432=EDGE_CURVE ( 'NONE', #5265, #833, #13114, .T. ) ;
#4438=AXIS2_PLACEMENT_3D ( 'NONE', #15437, #12034, #19305 ) ;
#4443=CARTESIAN_POINT ( 'NONE',  ( 12.69999999999999929, -3599.497499999999945, 2263.571799999999712 ) ) ;
#4449=ORIENTED_EDGE ( 'NONE', *, *, #2579, .T. ) ;
#4453=DIRECTION ( 'NONE',  ( 0.000000000000000000, 0.000000000000000000, 1.000000000000000000 ) ) ;
#4507=DIRECTION ( 'NONE',  ( 0.7071067811865969777, 0.000000000000000000, -0.7071067811864980568 ) ) ;
#4508=EDGE_CURVE ( 'NONE', #10059, #19085, #22071, .T. ) ;
#4509=ORIENTED_EDGE ( 'NONE', *, *, #22542, .F. ) ;
#4525=DIRECTION ( 'NONE',  ( 1.000000000000000000, 0.000000000000000000, 0.000000000000000000 ) ) ;
#4528=ORIENTED_EDGE ( 'NONE', *, *, #17738, .F. ) ;
#4536=ORIENTED_EDGE ( 'NONE', *, *, #18405, .F. ) ;
#4542=EDGE_CURVE ( 'NONE', #9572, #12083, #6754, .T. ) ;
#4547=EDGE_CURVE ( 'NONE', #9227, #8952, #12737, .T. ) ;
#4571=AXIS2_PLACEMENT_3D ( 'NONE', #20864, #1281, #6580 ) ;
#4575=VECTOR ( 'NONE', #12036, 1000.000000000000000 ) ;
#4577=DIRECTION ( 'NONE',  ( 1.000000000000000000, 0.000000000000000000, 0.000000000000000000 ) ) ;
#4582=CARTESIAN_POINT ( 'NONE',  ( 12.69999999999999929, -3599.497499999999945, 2288.971800000000258 ) ) ;
#4616=VERTEX_POINT ( 'NONE', #12634 ) ;
#4627=ORIENTED_EDGE ( 'NONE', *, *, #5455, .T. ) ;
#4633=VERTEX_POINT ( 'NONE', #18017 ) ;
#4650=DIRECTION ( 'NONE',  ( -1.000000000000000000, 0.000000000000000000, 0.000000000000000000 ) ) ;
#4665=CYLINDRICAL_SURFACE ( 'NONE', #12856, 0.7619999999999294005 ) ;
#4675=EDGE_CURVE ( 'NONE', #1205, #2446, #10112, .T. ) ;
#4684=LINE ( 'NONE', #11835, #10327 ) ;
#4687=TOROIDAL_SURFACE ( 'NONE', #12555, 3.606799999999999784, 0.7620000000000000107 ) ;
#4699=VECTOR ( 'NONE', #21407, 1000.000000000000000 ) ;
#4708=ORIENTED_EDGE ( 'NONE', *, *, #11776, .T. ) ;
#4718=AXIS2_PLACEMENT_3D ( 'NONE', #2971, #10118, #17263 ) ;
#4745=CARTESIAN_POINT ( 'NONE',  ( 0.7620000000000000107, -3544.061999999999898, 2275.763800000000174 ) ) ;
#4756=CARTESIAN_POINT ( 'NONE',  ( 64.76999999999999602, -3694.938000000000102, 2286.368300000000090 ) ) ;
#4823=ORIENTED_EDGE ( 'NONE', *, *, #2098, .F. ) ;
#4833=AXIS2_PLACEMENT_3D ( 'NONE', #6054, #18345, #20343 ) ;
#4834=EDGE_CURVE ( 'NONE', #9191, #7405, #3959, .T. ) ;
#4863=DIRECTION ( 'NONE',  ( 1.000000000000000000, 0.000000000000000000, 0.000000000000000000 ) ) ;
#4877=LINE ( 'NONE', #15899, #10696 ) ;
#4882=CARTESIAN_POINT ( 'NONE',  ( 55.57575231171000496, -3544.061999999999898, 2275.763800000000174 ) ) ;
#4889=ORIENTED_EDGE ( 'NONE', *, *, #13444, .F. ) ;
#4896=LINE ( 'NONE', #17778, #21430 ) ;
#4922=VERTEX_POINT ( 'NONE', #4756 ) ;
#4923=CYLINDRICAL_SURFACE ( 'NONE', #20127, 0.7619999999998802176 ) ;
#4938=EDGE_CURVE ( 'NONE', #19085, #4104, #20808, .T. ) ;
#4939=CARTESIAN_POINT ( 'NONE',  ( 64.76999999999999602, -3568.700000000000273, 2292.057900000000245 ) ) ;
#4950=CARTESIAN_POINT ( 'NONE',  ( 22.54063073453000143, -3694.938000000000102, 2275.763800000000174 ) ) ;
#4956=CIRCLE ( 'NONE', #21789, 2.844799999999999773 ) ;
#4969=FACE_OUTER_BOUND ( 'NONE', #20069, .T. ) ;
#4972=CARTESIAN_POINT ( 'NONE',  ( 20.32000000000000028, -3670.300000000000182, 2289.213099999999940 ) ) ;
#4976=CARTESIAN_POINT ( 'NONE',  ( 152.4000000000000057, -3544.061999999999898, 2275.763800000000174 ) ) ;
#4986=ORIENTED_EDGE ( 'NONE', *, *, #13454, .T. ) ;
#4992=ORIENTED_EDGE ( 'NONE', *, *, #18653, .T. ) ;
#4994=ADVANCED_FACE ( 'NONE', ( #3107 ), #10255, .T. ) ;
#5012=EDGE_LOOP ( 'NONE', ( #22238, #17207, #17566, #4310 ) ) ;
#5020=CARTESIAN_POINT ( 'NONE',  ( 0.7620000000000000107, -3544.061999999999898, 2296.591799999999694 ) ) ;
#5049=DIRECTION ( 'NONE',  ( 0.000000000000000000, 1.000000000000000000, 0.000000000000000000 ) ) ;
#5051=CARTESIAN_POINT ( 'NONE',  ( 0.7620000000000000107, -3544.061999999999898, 2296.591799999999694 ) ) ;
#5053=DIRECTION ( 'NONE',  ( 1.664719871139314556E-14, -1.000000000000000000, 0.000000000000000000 ) ) ;
#5057=CARTESIAN_POINT ( 'NONE',  ( 22.54063073453000143, -3694.938000000000102, 2275.763800000000174 ) ) ;
#5092=ORIENTED_EDGE ( 'NONE', *, *, #16140, .F. ) ;
#5100=VERTEX_POINT ( 'NONE', #21394 ) ;
#5111=EDGE_CURVE ( 'NONE', #4017, #8952, #13081, .T. ) ;
#5127=EDGE_LOOP ( 'NONE', ( #14291, #1496, #834, #1537 ) ) ;
#5134=DIRECTION ( 'NONE',  ( 0.000000000000000000, 1.000000000000000000, 0.000000000000000000 ) ) ;
#5137=AXIS2_PLACEMENT_3D ( 'NONE', #16675, #18436, #20426 ) ;
#5143=DIRECTION ( 'NONE',  ( 0.000000000000000000, 0.000000000000000000, 1.000000000000000000 ) ) ;
#5149=EDGE_CURVE ( 'NONE', #10742, #5531, #12716, .T. ) ;
#5150=CARTESIAN_POINT ( 'NONE',  ( 18.41499999999999915, -3639.502500000000055, 2288.971800000000258 ) ) ;
#5158=VECTOR ( 'NONE', #4577, 1000.000000000000000 ) ;
#5165=ADVANCED_FACE ( 'NONE', ( #14711 ), #20211, .F. ) ;
#5169=CARTESIAN_POINT ( 'NONE',  ( 20.32000000000000028, -3695.699999999999818, 2292.819899999999961 ) ) ;
#5171=CIRCLE ( 'NONE', #11503, 2.844800000000091700 ) ;
#5176=DIRECTION ( 'NONE',  ( 2.760304743598521628E-14, 1.000000000000000000, 0.000000000000000000 ) ) ;
#5182=LINE ( 'NONE', #20882, #18461 ) ;
#5196=DIRECTION ( 'NONE',  ( 0.000000000000000000, 0.000000000000000000, -1.000000000000000000 ) ) ;
#5209=VERTEX_POINT ( 'NONE', #3689 ) ;
#5216=EDGE_CURVE ( 'NONE', #5209, #9879, #21261, .T. ) ;
#5228=DIRECTION ( 'NONE',  ( 1.000000000000000000, 0.000000000000000000, 0.000000000000000000 ) ) ;
#5245=ORIENTED_EDGE ( 'NONE', *, *, #7034, .T. ) ;
#5257=CYLINDRICAL_SURFACE ( 'NONE', #21121, 0.7620000000000000107 ) ;
#5265=VERTEX_POINT ( 'NONE', #11876 ) ;
#5301=CARTESIAN_POINT ( 'NONE',  ( 20.32000000000000028, -3694.938000000000102, 2289.213099999999940 ) ) ;
#5305=CIRCLE ( 'NONE', #18392, 6.476999999999001112 ) ;
#5308=TOROIDAL_SURFACE ( 'NONE', #15402, 1.524000000000000021, 0.7620000000000000107 ) ;
#5311=VERTEX_POINT ( 'NONE', #11625 ) ;
#5315=CARTESIAN_POINT ( 'NONE',  ( 64.76999999999999602, -3670.300000000000182, 2292.057900000000245 ) ) ;
#5317=ORIENTED_EDGE ( 'NONE', *, *, #1795, .T. ) ;
#5329=DIRECTION ( 'NONE',  ( 1.000000000000000000, 0.000000000000000000, 0.000000000000000000 ) ) ;
#5341=AXIS2_PLACEMENT_3D ( 'NONE', #6664, #15675, #15908 ) ;
#5344=CARTESIAN_POINT ( 'NONE',  ( 20.32000000000000028, -3695.699999999999818, 2289.213099999999940 ) ) ;
#5345=EDGE_LOOP ( 'NONE', ( #14443, #1069, #16666, #7151 ) ) ;
#5357=AXIS2_PLACEMENT_3D ( 'NONE', #1574, #21156, #8734 ) ;
#5363=CARTESIAN_POINT ( 'NONE',  ( 64.76999999999999602, -3695.699999999999818, 2289.213099999999940 ) ) ;
#5367=DIRECTION ( 'NONE',  ( 0.000000000000000000, 1.000000000000000000, 0.000000000000000000 ) ) ;
#5372=EDGE_CURVE ( 'NONE', #1484, #11029, #6381, .T. ) ;
#5373=DIRECTION ( 'NONE',  ( 0.000000000000000000, 0.000000000000000000, 1.000000000000000000 ) ) ;
#5392=ORIENTED_EDGE ( 'NONE', *, *, #12284, .F. ) ;
#5412=FACE_OUTER_BOUND ( 'NONE', #19210, .T. ) ;
#5415=CARTESIAN_POINT ( 'NONE',  ( 12.69999999999999929, -3639.502500000000055, 2288.971800000000258 ) ) ;
#5455=EDGE_CURVE ( 'NONE', #7940, #6734, #20250, .T. ) ;
#5465=DIRECTION ( 'NONE',  ( 0.000000000000000000, 1.000000000000000000, 0.000000000000000000 ) ) ;
#5474=AXIS2_PLACEMENT_3D ( 'NONE', #22814, #6902, #6785 ) ;
#5475=FACE_OUTER_BOUND ( 'NONE', #17032, .T. ) ;
#5481=AXIS2_PLACEMENT_3D ( 'NONE', #17283, #2759, #22676 ) ;
#5483=AXIS2_PLACEMENT_3D ( 'NONE', #11950, #12064, #3039 ) ;
#5496=DIRECTION ( 'NONE',  ( 3.369279192186236859E-13, -1.000000000000000000, -5.827942386484301240E-13 ) ) ;
#5531=VERTEX_POINT ( 'NONE', #7270 ) ;
#5540=ORIENTED_EDGE ( 'NONE', *, *, #17533, .F. ) ;
#5553=CYLINDRICAL_SURFACE ( 'NONE', #649, 0.7619999999999294005 ) ;
#5561=AXIS2_PLACEMENT_3D ( 'NONE', #1409, #10549, #15601 ) ;
#5566=ORIENTED_EDGE ( 'NONE', *, *, #17727, .T. ) ;
#5573=PLANE ( 'NONE',  #22060 ) ;
#5600=DIRECTION ( 'NONE',  ( 0.000000000000000000, 0.000000000000000000, -1.000000000000000000 ) ) ;
#5611=AXIS2_PLACEMENT_3D ( 'NONE', #2606, #9751, #7545 ) ;
#5614=CYLINDRICAL_SURFACE ( 'NONE', #16266, 0.7619999999999294005 ) ;
#5617=CYLINDRICAL_SURFACE ( 'NONE', #12577, 5.715000000000001634 ) ;
#5619=ORIENTED_EDGE ( 'NONE', *, *, #12505, .F. ) ;
#5629=CARTESIAN_POINT ( 'NONE',  ( 6.223000000000999066, -3599.497499999999945, 2296.591799999999694 ) ) ;
#5633=CARTESIAN_POINT ( 'NONE',  ( 0.7620000000000000107, -3695.699999999999818, 2275.763800000000174 ) ) ;
#5646=DIRECTION ( 'NONE',  ( 0.000000000000000000, 0.000000000000000000, -1.000000000000000000 ) ) ;
#5647=VERTEX_POINT ( 'NONE', #22016 ) ;
#5649=CARTESIAN_POINT ( 'NONE',  ( 64.76999999999999602, -3670.300000000000182, 2289.213099999999940 ) ) ;
#5681=ORIENTED_EDGE ( 'NONE', *, *, #21985, .T. ) ;
#5701=DIRECTION ( 'NONE',  ( 1.000000000000000000, 0.000000000000000000, 0.000000000000000000 ) ) ;
#5703=ORIENTED_EDGE ( 'NONE', *, *, #9981, .F. ) ;
#5706=CYLINDRICAL_SURFACE ( 'NONE', #6590, 2.844800000000091700 ) ;
#5748=UNCERTAINTY_MEASURE_WITH_UNIT (LENGTH_MEASURE( 1.000000000000000082E-05 ), #9985, 'distance_accuracy_value', 'NONE');
#5765=FACE_OUTER_BOUND ( 'NONE', #9925, .T. ) ;
#5786=ORIENTED_EDGE ( 'NONE', *, *, #1509, .F. ) ;
#5799=CARTESIAN_POINT ( 'NONE',  ( 0.7620000000000000107, -3694.938000000000102, 2275.763800000000174 ) ) ;
#5804=DIRECTION ( 'NONE',  ( -1.224646799147353207E-16, 1.000000000000000000, 0.000000000000000000 ) ) ;
#5808=ORIENTED_EDGE ( 'NONE', *, *, #6706, .T. ) ;
#5821=CARTESIAN_POINT ( 'NONE',  ( 55.57575231171000496, -3544.061999999999898, 2275.763800000000174 ) ) ;
#5828=DIRECTION ( 'NONE',  ( 0.000000000000000000, 0.000000000000000000, 1.000000000000000000 ) ) ;
#5849=AXIS2_PLACEMENT_3D ( 'NONE', #4443, #11579, #915 ) ;
#5866=LINE ( 'NONE', #789, #2913 ) ;
#5878=CIRCLE ( 'NONE', #3232, 0.7619999999999987894 ) ;
#5888=DIRECTION ( 'NONE',  ( -1.000000000000000000, 0.000000000000000000, 0.000000000000000000 ) ) ;
#5891=DIRECTION ( 'NONE',  ( 0.000000000000000000, 0.000000000000000000, 1.000000000000000000 ) ) ;
#5920=LINE ( 'NONE', #1814, #8882 ) ;
#5941=CARTESIAN_POINT ( 'NONE',  ( 9.394261469291061317, -3543.299999999916054, 2281.667430734604750 ) ) ;
#5946=CARTESIAN_POINT ( 'NONE',  ( 20.32000000000000028, -3568.700000000000273, 2286.368300000000090 ) ) ;
#5953=ORIENTED_EDGE ( 'NONE', *, *, #9138, .T. ) ;
#5957=LINE ( 'NONE', #20570, #12148 ) ;
#5960=DIRECTION ( 'NONE',  ( 0.000000000000000000, 0.000000000000000000, -1.000000000000000000 ) ) ;
#5969=ORIENTED_EDGE ( 'NONE', *, *, #5216, .F. ) ;
#5975=AXIS2_PLACEMENT_3D ( 'NONE', #15322, #1013, #8288 ) ;
#5993=ORIENTED_EDGE ( 'NONE', *, *, #6250, .T. ) ;
#6003=CIRCLE ( 'NONE', #13461, 0.7619999999999683693 ) ;
#6004=CARTESIAN_POINT ( 'NONE',  ( 60.21459350832999746, -3543.299999999999727, 2280.170699136999701 ) ) ;
#6035=AXIS2_PLACEMENT_3D ( 'NONE', #17156, #6863, #6745 ) ;
#6054=CARTESIAN_POINT ( 'NONE',  ( 151.4000000000000057, -3694.938000000000102, 2295.829799999999977 ) ) ;
#6058=CARTESIAN_POINT ( 'NONE',  ( 16.19063073453000001, -3695.699999999999818, 2282.113800000000083 ) ) ;
#6061=EDGE_CURVE ( 'NONE', #14108, #4104, #18999, .T. ) ;
#6063=VECTOR ( 'NONE', #403, 1000.000000000000000 ) ;
#6065=CARTESIAN_POINT ( 'NONE',  ( 16.19063073453000001, -3695.699999999999818, 2282.113800000000083 ) ) ;
#6067=ORIENTED_EDGE ( 'NONE', *, *, #5111, .F. ) ;
#6070=EDGE_LOOP ( 'NONE', ( #1222, #21647 ) ) ;
#6099=CIRCLE ( 'NONE', #1978, 0.7619999999999294005 ) ;
#6105=EDGE_CURVE ( 'NONE', #18286, #18510, #17484, .T. ) ;
#6106=DIRECTION ( 'NONE',  ( 0.000000000000000000, 1.000000000000000000, 0.000000000000000000 ) ) ;
#6115=CIRCLE ( 'NONE', #852, 3.606800000000021100 ) ;
#6119=VERTEX_POINT ( 'NONE', #7584 ) ;
#6137=CARTESIAN_POINT ( 'NONE',  ( 61.26424768829000556, -3544.061999999999898, 2280.589800000000196 ) ) ;
#6164=CARTESIAN_POINT ( 'NONE',  ( 151.6380000000000052, -3543.299999999999727, 2295.829799999999977 ) ) ;
#6177=EDGE_LOOP ( 'NONE', ( #1631, #8717, #15513, #19488 ) ) ;
#6181=FACE_BOUND ( 'NONE', #1047, .T. ) ;
#6213=ADVANCED_FACE ( 'NONE', ( #11546 ), #18814, .F. ) ;
#6220=CIRCLE ( 'NONE', #9213, 2.844800000000091700 ) ;
#6249=VERTEX_POINT ( 'NONE', #6407 ) ;
#6250=EDGE_CURVE ( 'NONE', #11029, #4616, #4413, .T. ) ;
#6259=( NAMED_UNIT ( * ) SI_UNIT ( $, .STERADIAN. ) SOLID_ANGLE_UNIT ( ) );
#6266=DIRECTION ( 'NONE',  ( 0.000000000000000000, 0.000000000000000000, -1.000000000000000000 ) ) ;
#6270=ORIENTED_EDGE ( 'NONE', *, *, #7385, .T. ) ;
#6290=VERTEX_POINT ( 'NONE', #10612 ) ;
#6292=CIRCLE ( 'NONE', #23110, 3.606800000000021100 ) ;
#6302=FACE_OUTER_BOUND ( 'NONE', #17463, .T. ) ;
#6303=DIRECTION ( 'NONE',  ( 0.000000000000000000, 0.000000000000000000, -1.000000000000000000 ) ) ;
#6320=DIRECTION ( 'NONE',  ( 0.000000000000000000, 0.000000000000000000, -1.000000000000000000 ) ) ;
#6327=DIRECTION ( 'NONE',  ( 0.000000000000000000, 1.000000000000000000, 0.000000000000000000 ) ) ;
#6353=VECTOR ( 'NONE', #11544, 1000.000000000000000 ) ;
#6359=ORIENTED_EDGE ( 'NONE', *, *, #5111, .T. ) ;
#6363=ORIENTED_EDGE ( 'NONE', *, *, #1847, .T. ) ;
#6365=DIRECTION ( 'NONE',  ( 0.000000000000000000, 1.000000000000000000, 5.827942386484301240E-13 ) ) ;
#6374=ADVANCED_FACE ( 'NONE', ( #8746 ), #23050, .T. ) ;
#6379=EDGE_CURVE ( 'NONE', #1414, #1200, #20819, .T. ) ;
#6381=LINE ( 'NONE', #9874, #4409 ) ;
#6397=ORIENTED_EDGE ( 'NONE', *, *, #19335, .T. ) ;
#6407=CARTESIAN_POINT ( 'NONE',  ( 64.76999999999999602, -3694.938000000000102, 2292.057900000000245 ) ) ;
#6413=ORIENTED_EDGE ( 'NONE', *, *, #20193, .T. ) ;
#6417=ORIENTED_EDGE ( 'NONE', *, *, #16738, .T. ) ;
#6425=ORIENTED_EDGE ( 'NONE', *, *, #4834, .F. ) ;
#6496=EDGE_LOOP ( 'NONE', ( #15660, #13233, #7820, #18933 ) ) ;
#6502=CYLINDRICAL_SURFACE ( 'NONE', #4718, 0.7619999999999294005 ) ;
#6536=ORIENTED_EDGE ( 'NONE', *, *, #4432, .T. ) ;
#6538=AXIS2_PLACEMENT_3D ( 'NONE', #8045, #13547, #15197 ) ;
#6551=DIRECTION ( 'NONE',  ( 0.000000000000000000, -1.000000000000000000, 0.000000000000000000 ) ) ;
#6556=AXIS2_PLACEMENT_3D ( 'NONE', #18449, #15057, #743 ) ;
#6568=ORIENTED_EDGE ( 'NONE', *, *, #8238, .F. ) ;
#6580=DIRECTION ( 'NONE',  ( 1.000000000000000000, 0.000000000000000000, 0.000000000000000000 ) ) ;
#6589=ORIENTED_EDGE ( 'NONE', *, *, #16954, .T. ) ;
#6590=AXIS2_PLACEMENT_3D ( 'NONE', #191, #18226, #1832 ) ;
#6602=EDGE_LOOP ( 'NONE', ( #4992, #22313, #10953, #651 ) ) ;
#6616=CARTESIAN_POINT ( 'NONE',  ( 56.10057940169000545, -3694.938000000000102, 2275.211350432000472 ) ) ;
#6639=EDGE_LOOP ( 'NONE', ( #23127, #4215, #602, #10794 ) ) ;
#6664=CARTESIAN_POINT ( 'NONE',  ( 12.69999999999999929, -3639.502500000000055, 2263.571799999999712 ) ) ;
#6669=DIRECTION ( 'NONE',  ( 0.000000000000000000, 0.000000000000000000, -1.000000000000000000 ) ) ;
#6692=PRODUCT_DEFINITION_CONTEXT ( 'detailed design', #1255, 'design' ) ;
#6694=LINE ( 'NONE', #22831, #3978 ) ;
#6706=EDGE_CURVE ( 'NONE', #13565, #6249, #14107, .T. ) ;
#6709=EDGE_LOOP ( 'NONE', ( #22356, #8668, #6737, #20906 ) ) ;
#6711=SPHERICAL_SURFACE ( 'NONE', #15838, 0.7620000000000000107 ) ;
#6730=VERTEX_POINT ( 'NONE', #1321 ) ;
#6734=VERTEX_POINT ( 'NONE', #14221 ) ;
#6737=ORIENTED_EDGE ( 'NONE', *, *, #5372, .T. ) ;
#6745=DIRECTION ( 'NONE',  ( 1.000000000000000000, 0.000000000000000000, 0.000000000000000000 ) ) ;
#6750=ADVANCED_FACE ( 'NONE', ( #10463 ), #21021, .T. ) ;
#6754=CIRCLE ( 'NONE', #20231, 0.7619999999999294005 ) ;
#6766=FACE_OUTER_BOUND ( 'NONE', #8200, .T. ) ;
#6772=DIRECTION ( 'NONE',  ( 1.000000000000000000, 4.198251155732999970E-13, 0.000000000000000000 ) ) ;
#6773=CARTESIAN_POINT ( 'NONE',  ( 55.57575231171000496, -3694.938000000000102, 2275.763800000000174 ) ) ;
#6785=DIRECTION ( 'NONE',  ( 1.000000000000000000, 0.000000000000000000, 0.000000000000000000 ) ) ;
#6791=VERTEX_POINT ( 'NONE', #21488 ) ;
#6798=AXIS2_PLACEMENT_3D ( 'NONE', #10753, #5367, #90 ) ;
#6813=CARTESIAN_POINT ( 'NONE',  ( 0.7620000000000000107, -3544.061999999999898, 2275.763800000000174 ) ) ;
#6824=DIRECTION ( 'NONE',  ( 0.000000000000000000, 0.000000000000000000, -1.000000000000000000 ) ) ;
#6829=DIRECTION ( 'NONE',  ( -1.000000000000000000, 0.000000000000000000, 0.000000000000000000 ) ) ;
#6837=CARTESIAN_POINT ( 'NONE',  ( 12.69999999999999929, -3639.502500000000055, 2263.571799999999712 ) ) ;
#6846=ORIENTED_EDGE ( 'NONE', *, *, #20293, .F. ) ;
#6847=AXIS2_PLACEMENT_3D ( 'NONE', #1690, #14008, #22890 ) ;
#6850=ORIENTED_EDGE ( 'NONE', *, *, #8235, .F. ) ;
#6863=DIRECTION ( 'NONE',  ( 0.000000000000000000, 0.000000000000000000, -1.000000000000000000 ) ) ;
#6884=ADVANCED_FACE ( 'NONE', ( #15031 ), #8339, .F. ) ;
#6893=DIRECTION ( 'NONE',  ( 0.000000000000000000, 0.000000000000000000, -1.000000000000000000 ) ) ;
#6894=AXIS2_PLACEMENT_3D ( 'NONE', #3632, #8572, #8683 ) ;
#6902=DIRECTION ( 'NONE',  ( 0.000000000000000000, 0.000000000000000000, 1.000000000000000000 ) ) ;
#6916=FACE_BOUND ( 'NONE', #14347, .T. ) ;
#6940=TOROIDAL_SURFACE ( 'NONE', #13277, 3.606799999999999784, 0.7620000000000000107 ) ;
#6947=CARTESIAN_POINT ( 'NONE',  ( 64.76999999999999602, -3670.300000000000182, 2292.057900000000245 ) ) ;
#6953=DIRECTION ( 'NONE',  ( -1.752935795934731214E-12, -1.000000000000000000, -1.748382715945290473E-12 ) ) ;
#6955=DIRECTION ( 'NONE',  ( -1.000000000000000000, 0.000000000000000000, 0.000000000000000000 ) ) ;
#6968=AXIS2_PLACEMENT_3D ( 'NONE', #12221, #22400, #3307 ) ;
#6969=ORIENTED_EDGE ( 'NONE', *, *, #7361, .F. ) ;
#6970=ORIENTED_EDGE ( 'NONE', *, *, #6250, .F. ) ;
#6972=ORIENTED_EDGE ( 'NONE', *, *, #22811, .T. ) ;
#6980=ORIENTED_EDGE ( 'NONE', *, *, #11576, .F. ) ;
#6984=CYLINDRICAL_SURFACE ( 'NONE', #5357, 0.7619999999999230722 ) ;
#7005=DIRECTION ( 'NONE',  ( 0.000000000000000000, 1.000000000000000000, 0.000000000000000000 ) ) ;
#7018=ORIENTED_EDGE ( 'NONE', *, *, #18653, .F. ) ;
#7034=EDGE_CURVE ( 'NONE', #12115, #19405, #19691, .T. ) ;
#7045=EDGE_LOOP ( 'NONE', ( #12444, #12465 ) ) ;
#7053=CARTESIAN_POINT ( 'NONE',  ( 15.54479999999999862, -3639.502500000000055, 2281.351799999999912 ) ) ;
#7069=EDGE_CURVE ( 'NONE', #22409, #11834, #22644, .T. ) ;
#7072=EDGE_CURVE ( 'NONE', #18510, #5531, #23034, .T. ) ;
#7091=CARTESIAN_POINT ( 'NONE',  ( 0.000000000000000000, -3544.061999999999898, 2275.763800000000174 ) ) ;
#7096=ORIENTED_EDGE ( 'NONE', *, *, #2924, .T. ) ;
#7106=EDGE_CURVE ( 'NONE', #9540, #12400, #11066, .T. ) ;
#7111=DIRECTION ( 'NONE',  ( 0.6887494619136477203, 0.000000000000000000, -0.7249994335954068614 ) ) ;
#7128=EDGE_CURVE ( 'NONE', #4922, #13263, #14087, .T. ) ;
#7132=CARTESIAN_POINT ( 'NONE',  ( 12.69999999999999929, -3599.497499999999945, 2281.351799999999912 ) ) ;
#7148=VERTEX_POINT ( 'NONE', #14145 ) ;
#7151=ORIENTED_EDGE ( 'NONE', *, *, #6061, .F. ) ;
#7165=CARTESIAN_POINT ( 'NONE',  ( 64.76999999999999602, -3544.061999999999898, 2292.057900000000245 ) ) ;
#7168=DIRECTION ( 'NONE',  ( 0.000000000000000000, 0.000000000000000000, -1.000000000000000000 ) ) ;
#7189=DIRECTION ( 'NONE',  ( 0.000000000000000000, 1.000000000000000000, 0.000000000000000000 ) ) ;
#7192=ORIENTED_EDGE ( 'NONE', *, *, #7928, .T. ) ;
#7222=DIRECTION ( 'NONE',  ( 0.000000000000000000, 1.000000000000000000, 0.000000000000000000 ) ) ;
#7270=CARTESIAN_POINT ( 'NONE',  ( 0.000000000000000000, -3544.061999999999898, 2295.829799999999977 ) ) ;
#7276=LINE ( 'NONE', #14200, #927 ) ;
#7284=CARTESIAN_POINT ( 'NONE',  ( 151.4000000000000057, -3544.061999999999898, 2296.591799999999694 ) ) ;
#7300=DIRECTION ( 'NONE',  ( 0.000000000000000000, 0.000000000000000000, 1.000000000000000000 ) ) ;
#7304=ORIENTED_EDGE ( 'NONE', *, *, #17687, .T. ) ;
#7309=AXIS2_PLACEMENT_3D ( 'NONE', #5415, #22571, #4650 ) ;
#7321=FACE_OUTER_BOUND ( 'NONE', #15142, .T. ) ;
#7328=ORIENTED_EDGE ( 'NONE', *, *, #12505, .T. ) ;
#7334=ORIENTED_EDGE ( 'NONE', *, *, #3052, .F. ) ;
#7338=CARTESIAN_POINT ( 'NONE',  ( 64.76999999999999602, -3568.700000000000273, 2289.213099999999940 ) ) ;
#7357=FACE_OUTER_BOUND ( 'NONE', #13844, .T. ) ;
#7359=DIRECTION ( 'NONE',  ( 0.000000000000000000, 0.000000000000000000, 1.000000000000000000 ) ) ;
#7361=EDGE_CURVE ( 'NONE', #1371, #10059, #10104, .T. ) ;
#7368=CYLINDRICAL_SURFACE ( 'NONE', #15865, 0.7619999999999294005 ) ;
#7375=EDGE_LOOP ( 'NONE', ( #5317, #16502, #22269, #3085 ) ) ;
#7385=EDGE_CURVE ( 'NONE', #10237, #3900, #15575, .T. ) ;
#7402=ORIENTED_EDGE ( 'NONE', *, *, #20299, .T. ) ;
#7405=VERTEX_POINT ( 'NONE', #8589 ) ;
#7408=DIRECTION ( 'NONE',  ( 0.6887494619135663410, 0.000000000000000000, -0.7249994335954840219 ) ) ;
#7418=DIRECTION ( 'NONE',  ( 0.000000000000000000, 0.000000000000000000, -1.000000000000000000 ) ) ;
#7421=EDGE_CURVE ( 'NONE', #11162, #19328, #11742, .T. ) ;
#7432=CARTESIAN_POINT ( 'NONE',  ( 22.54063073453000143, -3694.938000000000102, 2275.001800000000003 ) ) ;
#7434=ORIENTED_EDGE ( 'NONE', *, *, #4547, .F. ) ;
#7435=DIRECTION ( 'NONE',  ( 0.000000000000000000, 1.000000000000000000, 0.000000000000000000 ) ) ;
#7466=DIRECTION ( 'NONE',  ( 0.000000000000000000, 0.000000000000000000, 1.000000000000000000 ) ) ;
#7474=ORIENTED_EDGE ( 'NONE', *, *, #6379, .T. ) ;
#7475=CARTESIAN_POINT ( 'NONE',  ( 12.69999999999999929, -3599.497499999999945, 2288.971800000000258 ) ) ;
#7485=PRODUCT_DEFINITION_FORMATION_WITH_SPECIFIED_SOURCE ( 'ANY', '', #15546, .NOT_KNOWN. ) ;
#7489=CARTESIAN_POINT ( 'NONE',  ( 9.525000000091798924, -3694.938000000000102, 2281.351800000090861 ) ) ;
#7504=ORIENTED_EDGE ( 'NONE', *, *, #20973, .F. ) ;
#7535=DIRECTION ( 'NONE',  ( -1.000000000000000000, 0.000000000000000000, 0.000000000000000000 ) ) ;
#7539=DIRECTION ( 'NONE',  ( 1.000000000000000000, 0.000000000000000000, 0.000000000000000000 ) ) ;
#7542=CIRCLE ( 'NONE', #15776, 5.714999999999999858 ) ;
#7543=EDGE_CURVE ( 'NONE', #3230, #22365, #21006, .T. ) ;
#7545=DIRECTION ( 'NONE',  ( 1.000000000000000000, 0.000000000000000000, 0.000000000000000000 ) ) ;
#7547=DIRECTION ( 'NONE',  ( -1.000000000000000000, 0.000000000000000000, 0.000000000000000000 ) ) ;
#7549=CARTESIAN_POINT ( 'NONE',  ( 56.10057940169000545, -3544.061999999999898, 2275.211350432000472 ) ) ;
#7551=FACE_OUTER_BOUND ( 'NONE', #9609, .T. ) ;
#7552=DIRECTION ( 'NONE',  ( 0.7071067811864976127, 0.000000000000000000, 0.7071067811865975328 ) ) ;
#7560=CYLINDRICAL_SURFACE ( 'NONE', #13733, 2.844800000000091700 ) ;
#7563=EDGE_LOOP ( 'NONE', ( #17629, #3166, #13129, #21802 ) ) ;
#7577=VECTOR ( 'NONE', #18261, 1000.000000000000000 ) ;
#7584=CARTESIAN_POINT ( 'NONE',  ( 55.57575231171000496, -3694.938000000000102, 2275.001800000000003 ) ) ;
#7586=CARTESIAN_POINT ( 'NONE',  ( 55.57575231171000496, -3694.938000000000102, 2275.763800000000174 ) ) ;
#7606=CARTESIAN_POINT ( 'NONE',  ( 64.76999999999999602, -3694.938000000000102, 2289.213099999999940 ) ) ;
#7609=FACE_OUTER_BOUND ( 'NONE', #20444, .T. ) ;
#7613=ORIENTED_EDGE ( 'NONE', *, *, #22514, .F. ) ;
#7629=CARTESIAN_POINT ( 'NONE',  ( 64.76999999999999602, -3568.700000000000273, 2289.213099999999940 ) ) ;
#7632=ADVANCED_FACE ( 'NONE', ( #19828, #12788, #1658 ), #19945, .F. ) ;
#7634=ORIENTED_EDGE ( 'NONE', *, *, #8356, .F. ) ;
#7643=CARTESIAN_POINT ( 'NONE',  ( 0.7620000000000000107, -3544.061999999999898, 2295.829799999999977 ) ) ;
#7650=DIRECTION ( 'NONE',  ( 0.000000000000000000, 1.000000000000000000, 0.000000000000000000 ) ) ;
#7658=CARTESIAN_POINT ( 'NONE',  ( 25.98329380356999962, -3544.061999999999898, 2247.650964417000068 ) ) ;
#7661=EDGE_CURVE ( 'NONE', #19085, #3900, #15367, .T. ) ;
#7662=CIRCLE ( 'NONE', #14401, 0.7620000000000366480 ) ;
#7671=ADVANCED_BREP_SHAPE_REPRESENTATION ( '', ( #13285, #5611 ), #15735 ) ;
#7695=ORIENTED_EDGE ( 'NONE', *, *, #14636, .T. ) ;
#7702=CIRCLE ( 'NONE', #17750, 5.714999999998999769 ) ;
#7718=ORIENTED_EDGE ( 'NONE', *, *, #1509, .T. ) ;
#7731=AXIS2_PLACEMENT_3D ( 'NONE', #23022, #5465, #17991 ) ;
#7733=CIRCLE ( 'NONE', #20822, 2.844800000000091700 ) ;
#7752=ORIENTED_EDGE ( 'NONE', *, *, #7798, .F. ) ;
#7777=CARTESIAN_POINT ( 'NONE',  ( 1.048684632737000300, -3544.061999999999898, 2273.953115367000009 ) ) ;
#7781=DIRECTION ( 'NONE',  ( 0.000000000000000000, -1.000000000000000000, 0.000000000000000000 ) ) ;
#7785=DIRECTION ( 'NONE',  ( 0.000000000000000000, -1.000000000000000000, 0.000000000000000000 ) ) ;
#7798=EDGE_CURVE ( 'NONE', #1742, #13263, #414, .T. ) ;
#7809=DIRECTION ( 'NONE',  ( 0.000000000000000000, 0.000000000000000000, 1.000000000000000000 ) ) ;
#7814=FACE_OUTER_BOUND ( 'NONE', #21871, .T. ) ;
#7820=ORIENTED_EDGE ( 'NONE', *, *, #2424, .T. ) ;
#7824=DIRECTION ( 'NONE',  ( 0.000000000000000000, -1.000000000000000000, 0.000000000000000000 ) ) ;
#7834=EDGE_CURVE ( 'NONE', #6249, #1742, #17714, .T. ) ;
#7876=ORIENTED_EDGE ( 'NONE', *, *, #6379, .F. ) ;
#7880=VERTEX_POINT ( 'NONE', #12970 ) ;
#7882=DIRECTION ( 'NONE',  ( -1.000000000000000000, 0.000000000000000000, 0.000000000000000000 ) ) ;
#7905=ORIENTED_EDGE ( 'NONE', *, *, #2098, .T. ) ;
#7915=DIRECTION ( 'NONE',  ( 0.000000000000000000, 0.000000000000000000, 1.000000000000000000 ) ) ;
#7924=CIRCLE ( 'NONE', #3437, 5.714999999999999858 ) ;
#7925=LINE ( 'NONE', #6065, #15064 ) ;
#7928=EDGE_CURVE ( 'NONE', #16884, #3779, #993, .T. ) ;
#7935=ORIENTED_EDGE ( 'NONE', *, *, #3283, .T. ) ;
#7940=VERTEX_POINT ( 'NONE', #4403 ) ;
#7953=ORIENTED_EDGE ( 'NONE', *, *, #12214, .F. ) ;
#7962=EDGE_CURVE ( 'NONE', #12400, #9540, #20315, .T. ) ;
#7967=FACE_OUTER_BOUND ( 'NONE', #7563, .T. ) ;
#7970=FACE_OUTER_BOUND ( 'NONE', #2985, .T. ) ;
#7988=DIRECTION ( 'NONE',  ( 1.000000000000000000, 0.000000000000000000, 0.000000000000000000 ) ) ;
#7994=EDGE_CURVE ( 'NONE', #19405, #12115, #3848, .T. ) ;
#8008=CARTESIAN_POINT ( 'NONE',  ( 19.17699999999900129, -3599.497499999999945, 2295.829799999999977 ) ) ;
#8009=( NAMED_UNIT ( * ) PLANE_ANGLE_UNIT ( ) SI_UNIT ( $, .RADIAN. ) );
#8029=DIRECTION ( 'NONE',  ( 0.000000000000000000, 1.000000000000000000, 0.000000000000000000 ) ) ;
#8045=CARTESIAN_POINT ( 'NONE',  ( 64.76999999999999602, -3544.061999999999898, 2289.213099999999940 ) ) ;
#8054=AXIS2_PLACEMENT_3D ( 'NONE', #5649, #10912, #9041 ) ;
#8089=ORIENTED_EDGE ( 'NONE', *, *, #2929, .F. ) ;
#8132=DIRECTION ( 'NONE',  ( -0.6887494619147132013, 0.000000000000000000, 0.7249994335943947821 ) ) ;
#8133=DIRECTION ( 'NONE',  ( 1.000000000000000000, 0.000000000000000000, 0.000000000000000000 ) ) ;
#8146=ORIENTED_EDGE ( 'NONE', *, *, #18717, .T. ) ;
#8147=ORIENTED_EDGE ( 'NONE', *, *, #18262, .T. ) ;
#8155=VERTEX_POINT ( 'NONE', #13778 ) ;
#8171=AXIS2_PLACEMENT_3D ( 'NONE', #6813, #5049, #22732 ) ;
#8197=PLANE ( 'NONE',  #2807 ) ;
#8200=EDGE_LOOP ( 'NONE', ( #4823, #14261, #12308, #2799 ) ) ;
#8204=ORIENTED_EDGE ( 'NONE', *, *, #7385, .F. ) ;
#8218=ADVANCED_FACE ( 'NONE', ( #3915 ), #21846, .T. ) ;
#8221=EDGE_CURVE ( 'NONE', #4633, #6290, #20880, .T. ) ;
#8222=ORIENTED_EDGE ( 'NONE', *, *, #7421, .T. ) ;
#8235=EDGE_CURVE ( 'NONE', #20799, #13309, #9080, .T. ) ;
#8238=EDGE_CURVE ( 'NONE', #5100, #12459, #1372, .T. ) ;
#8260=VERTEX_POINT ( 'NONE', #16112 ) ;
#8263=EDGE_CURVE ( 'NONE', #5209, #1371, #5920, .T. ) ;
#8288=DIRECTION ( 'NONE',  ( 1.000000000000000000, 0.000000000000000000, 0.000000000000000000 ) ) ;
#8295=AXIS2_PLACEMENT_3D ( 'NONE', #21352, #2950, #2012 ) ;
#8339=CYLINDRICAL_SURFACE ( 'NONE', #12942, 5.714999999998998881 ) ;
#8350=CARTESIAN_POINT ( 'NONE',  ( 161.1088462396999716, -3543.299999999999727, 2279.827800000000025 ) ) ;
#8356=EDGE_CURVE ( 'NONE', #9308, #22211, #15604, .T. ) ;
#8392=CARTESIAN_POINT ( 'NONE',  ( 15.87499999999605116, -3544.061999999999898, 2281.351799999999912 ) ) ;
#8401=CARTESIAN_POINT ( 'NONE',  ( 3.175000000003000089, -3544.061999999999898, 2275.001800000000003 ) ) ;
#8408=AXIS2_PLACEMENT_3D ( 'NONE', #16918, #654, #2526 ) ;
#8410=CARTESIAN_POINT ( 'NONE',  ( 15.54479999999999862, -3639.502500000000055, 2263.571799999999712 ) ) ;
#8469=CARTESIAN_POINT ( 'NONE',  ( 151.4000000000000057, -3543.299999999999727, 2295.829799999999977 ) ) ;
#8470=FACE_OUTER_BOUND ( 'NONE', #12777, .T. ) ;
#8472=CARTESIAN_POINT ( 'NONE',  ( 0.7620000000000000107, -3694.938000000000102, 2295.829799999999977 ) ) ;
#8477=DIRECTION ( 'NONE',  ( -0.7071067811865969777, 0.000000000000000000, -0.7071067811864980568 ) ) ;
#8489=ADVANCED_FACE ( 'NONE', ( #19134 ), #19366, .F. ) ;
#8491=CIRCLE ( 'NONE', #9249, 0.7619999999999294005 ) ;
#8512=DIRECTION ( 'NONE',  ( 0.000000000000000000, 1.000000000000000000, 0.000000000000000000 ) ) ;
#8516=EDGE_CURVE ( 'NONE', #3779, #6730, #8491, .T. ) ;
#8529=AXIS2_PLACEMENT_3D ( 'NONE', #13340, #18494, #6320 ) ;
#8535=ORIENTED_EDGE ( 'NONE', *, *, #2128, .F. ) ;
#8537=LINE ( 'NONE', #1482, #1972 ) ;
#8547=CARTESIAN_POINT ( 'NONE',  ( 152.4000000000000057, -3694.938000000000102, 2280.589800000000196 ) ) ;
#8548=DIRECTION ( 'NONE',  ( 0.000000000000000000, 0.000000000000000000, 1.000000000000000000 ) ) ;
#8557=EDGE_CURVE ( 'NONE', #9431, #7940, #2956, .T. ) ;
#8563=DIRECTION ( 'NONE',  ( -0.7249994335944036639, 0.000000000000000000, -0.6887494619147036534 ) ) ;
#8572=DIRECTION ( 'NONE',  ( 0.000000000000000000, 1.000000000000000000, 0.000000000000000000 ) ) ;
#8589=CARTESIAN_POINT ( 'NONE',  ( 15.87499999999605116, -3544.061999999999898, 2281.351799999999912 ) ) ;
#8606=DIRECTION ( 'NONE',  ( -0.7071067811865691111, 0.000000000000000000, 0.7071067811865258124 ) ) ;
#8643=CARTESIAN_POINT ( 'NONE',  ( 20.32000000000000028, -3543.299999999999727, 2292.819899999999961 ) ) ;
#8650=DIRECTION ( 'NONE',  ( 1.000000000000000000, 0.000000000000000000, 0.000000000000000000 ) ) ;
#8657=CARTESIAN_POINT ( 'NONE',  ( 0.7620000000000000107, -3544.061999999999898, 2275.001800000000003 ) ) ;
#8661=ORIENTED_EDGE ( 'NONE', *, *, #6105, .T. ) ;
#8668=ORIENTED_EDGE ( 'NONE', *, *, #9941, .F. ) ;
#8669=ORIENTED_EDGE ( 'NONE', *, *, #13042, .F. ) ;
#8675=CARTESIAN_POINT ( 'NONE',  ( 106.0884186392999879, -3694.938000000000102, 2323.750833010999941 ) ) ;
#8680=VECTOR ( 'NONE', #636, 1000.000000000000000 ) ;
#8683=DIRECTION ( 'NONE',  ( 0.000000000000000000, 0.000000000000000000, -1.000000000000000000 ) ) ;
#8691=DIRECTION ( 'NONE',  ( 0.000000000000000000, 1.000000000000000000, 0.000000000000000000 ) ) ;
#8717=ORIENTED_EDGE ( 'NONE', *, *, #20734, .T. ) ;
#8734=DIRECTION ( 'NONE',  ( 0.7071067811865691111, 0.000000000000000000, 0.7071067811865258124 ) ) ;
#8746=FACE_OUTER_BOUND ( 'NONE', #10693, .T. ) ;
#8747=VECTOR ( 'NONE', #4507, 1000.000000000000000 ) ;
#8754=ORIENTED_EDGE ( 'NONE', *, *, #22802, .F. ) ;
#8763=EDGE_LOOP ( 'NONE', ( #13879, #18506, #17793, #16697 ) ) ;
#8768=DIRECTION ( 'NONE',  ( -1.000000000000000000, -0.000000000000000000, -0.000000000000000000 ) ) ;
#8775=CARTESIAN_POINT ( 'NONE',  ( 0.7620000000000000107, -3694.938000000000102, 2275.001800000000003 ) ) ;
#8793=CARTESIAN_POINT ( 'NONE',  ( 22.54063073453000143, -3694.938000000000102, 2275.763800000000174 ) ) ;
#8810=EDGE_CURVE ( 'NONE', #13309, #5311, #16731, .T. ) ;
#8812=TOROIDAL_SURFACE ( 'NONE', #12171, 6.477000000000000313, 0.7620000000000000107 ) ;
#8828=ORIENTED_EDGE ( 'NONE', *, *, #14605, .T. ) ;
#8842=CARTESIAN_POINT ( 'NONE',  ( 3.175000000003000089, -3694.938000000000102, 2275.001800000000003 ) ) ;
#8846=ADVANCED_FACE ( 'NONE', ( #9505 ), #15130, .T. ) ;
#8864=CARTESIAN_POINT ( 'NONE',  ( 0.000000000000000000, -3695.699999999999818, 2275.001800000000003 ) ) ;
#8867=DIRECTION ( 'NONE',  ( 0.000000000000000000, 1.000000000000000000, 0.000000000000000000 ) ) ;
#8872=DIRECTION ( 'NONE',  ( 0.000000000000000000, 1.000000000000000000, 0.000000000000000000 ) ) ;
#8878=VERTEX_POINT ( 'NONE', #2367 ) ;
#8879=VECTOR ( 'NONE', #9026, 1000.000000000000000 ) ;
#8882=VECTOR ( 'NONE', #8965, 1000.000000000000000 ) ;
#8903=EDGE_LOOP ( 'NONE', ( #18187, #11530 ) ) ;
#8905=LINE ( 'NONE', #16617, #15103 ) ;
#8916=DIRECTION ( 'NONE',  ( 0.000000000000000000, -1.000000000000000000, 0.000000000000000000 ) ) ;
#8921=CARTESIAN_POINT ( 'NONE',  ( 152.4000000000000057, -3695.699999999999818, 2275.001800000000003 ) ) ;
#8929=CARTESIAN_POINT ( 'NONE',  ( 6.985000000000000320, -3639.502500000000055, 2288.971800000000258 ) ) ;
#8933=DIRECTION ( 'NONE',  ( 0.000000000000000000, -1.000000000000000000, 0.000000000000000000 ) ) ;
#8943=DIRECTION ( 'NONE',  ( 1.000000000000000000, 0.000000000000000000, 0.000000000000000000 ) ) ;
#8948=ADVANCED_FACE ( 'NONE', ( #3043 ), #4923, .T. ) ;
#8952=VERTEX_POINT ( 'NONE', #5169 ) ;
#8965=DIRECTION ( 'NONE',  ( 0.000000000000000000, 1.000000000000000000, 0.000000000000000000 ) ) ;
#8983=FACE_OUTER_BOUND ( 'NONE', #15986, .T. ) ;
#8987=CARTESIAN_POINT ( 'NONE',  ( 64.76999999999999602, -3694.938000000000102, 2292.819899999999961 ) ) ;
#9000=EDGE_CURVE ( 'NONE', #8155, #22365, #10529, .T. ) ;
#9026=DIRECTION ( 'NONE',  ( 0.000000000000000000, 0.000000000000000000, 1.000000000000000000 ) ) ;
#9029=DIRECTION ( 'NONE',  ( -1.000000000000000000, 2.760304743598999993E-14, 0.000000000000000000 ) ) ;
#9034=ORIENTED_EDGE ( 'NONE', *, *, #15973, .F. ) ;
#9041=DIRECTION ( 'NONE',  ( 0.000000000000000000, 0.000000000000000000, -1.000000000000000000 ) ) ;
#9060=ORIENTED_EDGE ( 'NONE', *, *, #2416, .T. ) ;
#9062=ORIENTED_EDGE ( 'NONE', *, *, #9935, .T. ) ;
#9076=ORIENTED_EDGE ( 'NONE', *, *, #7421, .F. ) ;
#9080=LINE ( 'NONE', #20095, #2502 ) ;
#9083=VERTEX_POINT ( 'NONE', #5629 ) ;
#9092=DIRECTION ( 'NONE',  ( -1.000000000000000000, -0.000000000000000000, -0.000000000000000000 ) ) ;
#9095=FACE_OUTER_BOUND ( 'NONE', #18518, .T. ) ;
#9096=CIRCLE ( 'NONE', #476, 0.7619999999999758078 ) ;
#9113=EDGE_LOOP ( 'NONE', ( #6536, #22727 ) ) ;
#9117=CIRCLE ( 'NONE', #21089, 0.7620000000000000107 ) ;
#9125=FACE_OUTER_BOUND ( 'NONE', #1778, .T. ) ;
#9138=EDGE_CURVE ( 'NONE', #3812, #14108, #5866, .T. ) ;
#9144=EDGE_CURVE ( 'NONE', #13263, #1742, #19007, .T. ) ;
#9160=DIRECTION ( 'NONE',  ( -1.000000000000000000, 0.000000000000000000, 0.000000000000000000 ) ) ;
#9182=VECTOR ( 'NONE', #20248, 1000.000000000000000 ) ;
#9191=VERTEX_POINT ( 'NONE', #20368 ) ;
#9201=AXIS2_PLACEMENT_3D ( 'NONE', #19298, #3237, #19061 ) ;
#9204=DIRECTION ( 'NONE',  ( -1.000000000000000000, 0.000000000000000000, 0.000000000000000000 ) ) ;
#9207=CARTESIAN_POINT ( 'NONE',  ( 15.54479999999999862, -3599.497499999999945, 2288.971800000000258 ) ) ;
#9213=AXIS2_PLACEMENT_3D ( 'NONE', #4421, #7824, #20358 ) ;
#9223=CARTESIAN_POINT ( 'NONE',  ( 12.69999999999999929, -3599.497499999999945, 2295.829799999999977 ) ) ;
#9227=VERTEX_POINT ( 'NONE', #11570 ) ;
#9236=DIRECTION ( 'NONE',  ( 0.000000000000000000, 0.000000000000000000, 1.000000000000000000 ) ) ;
#9248=AXIS2_PLACEMENT_3D ( 'NONE', #3659, #7300, #7988 ) ;
#9249=AXIS2_PLACEMENT_3D ( 'NONE', #4950, #3071, #6953 ) ;
#9269=ORIENTED_EDGE ( 'NONE', *, *, #14571, .F. ) ;
#9271=EDGE_CURVE ( 'NONE', #18622, #13565, #5171, .T. ) ;
#9284=DIRECTION ( 'NONE',  ( 0.7249994335955246560, 0.000000000000000000, 0.6887494619135237084 ) ) ;
#9292=CARTESIAN_POINT ( 'NONE',  ( 22.54063073453000143, -3543.299999999999727, 2275.763800000000174 ) ) ;
#9302=EDGE_CURVE ( 'NONE', #15238, #12083, #6292, .T. ) ;
#9305=ORIENTED_EDGE ( 'NONE', *, *, #12666, .F. ) ;
#9308=VERTEX_POINT ( 'NONE', #18013 ) ;
#9312=VERTEX_POINT ( 'NONE', #18127 ) ;
#9314=DIRECTION ( 'NONE',  ( 0.000000000000000000, 0.000000000000000000, 1.000000000000000000 ) ) ;
#9315=EDGE_CURVE ( 'NONE', #12115, #12400, #2534, .T. ) ;
#9335=VECTOR ( 'NONE', #9557, 1000.000000000000000 ) ;
#9366=ORIENTED_EDGE ( 'NONE', *, *, #1, .F. ) ;
#9385=DIRECTION ( 'NONE',  ( -1.000000000000000000, 0.000000000000000000, 0.000000000000000000 ) ) ;
#9411=ORIENTED_EDGE ( 'NONE', *, *, #7661, .T. ) ;
#9424=SPHERICAL_SURFACE ( 'NONE', #2491, 0.7620000000000000107 ) ;
#9431=VERTEX_POINT ( 'NONE', #17020 ) ;
#9433=EDGE_CURVE ( 'NONE', #11168, #7880, #17495, .T. ) ;
#9462=DIRECTION ( 'NONE',  ( -1.000000000000000000, 0.000000000000000000, 0.000000000000000000 ) ) ;
#9486=DIRECTION ( 'NONE',  ( 0.000000000000000000, 1.000000000000000000, 0.000000000000000000 ) ) ;
#9498=DIRECTION ( 'NONE',  ( -1.122008997397786234E-13, 0.000000000000000000, -1.000000000000000000 ) ) ;
#9501=DIRECTION ( 'NONE',  ( 0.000000000000000000, 1.000000000000000000, 0.000000000000000000 ) ) ;
#9503=CARTESIAN_POINT ( 'NONE',  ( 64.76999999999999602, -3694.938000000000102, 2289.213099999999940 ) ) ;
#9505=FACE_OUTER_BOUND ( 'NONE', #17120, .T. ) ;
#9514=EDGE_LOOP ( 'NONE', ( #9949, #7905, #616, #5392 ) ) ;
#9531=ADVANCED_FACE ( 'NONE', ( #16903 ), #11745, .T. ) ;
#9534=CARTESIAN_POINT ( 'NONE',  ( 9.209369265467998389, -3543.299999999999727, 2282.113800000000083 ) ) ;
#9540=VERTEX_POINT ( 'NONE', #2962 ) ;
#9554=TOROIDAL_SURFACE ( 'NONE', #3954, 3.606799999999999784, 0.7620000000000000107 ) ;
#9557=DIRECTION ( 'NONE',  ( -1.000000000000000000, 0.000000000000000000, 0.000000000000000000 ) ) ;
#9566=DIRECTION ( 'NONE',  ( 0.000000000000000000, 0.000000000000000000, 1.000000000000000000 ) ) ;
#9572=VERTEX_POINT ( 'NONE', #3427 ) ;
#9576=ORIENTED_EDGE ( 'NONE', *, *, #12076, .T. ) ;
#9577=AXIS2_PLACEMENT_3D ( 'NONE', #1770, #8916, #22963 ) ;
#9609=EDGE_LOOP ( 'NONE', ( #12326, #16192, #10967, #7504 ) ) ;
#9614=ORIENTED_EDGE ( 'NONE', *, *, #8810, .T. ) ;
#9636=PRODUCT_DEFINITION ( 'UNKNOWN', '', #7485, #6692 ) ;
#9639=ORIENTED_EDGE ( 'NONE', *, *, #10371, .T. ) ;
#9647=DIRECTION ( 'NONE',  ( 0.000000000000000000, 0.000000000000000000, -1.000000000000000000 ) ) ;
#9674=AXIS2_PLACEMENT_3D ( 'NONE', #4882, #6772, #18950 ) ;
#9701=EDGE_LOOP ( 'NONE', ( #18524, #10350, #22140, #13700 ) ) ;
#9720=VECTOR ( 'NONE', #7781, 1000.000000000000000 ) ;
#9724=EDGE_CURVE ( 'NONE', #8952, #4017, #19775, .T. ) ;
#9751=DIRECTION ( 'NONE',  ( 0.000000000000000000, 0.000000000000000000, 1.000000000000000000 ) ) ;
#9752=CARTESIAN_POINT ( 'NONE',  ( 61.26424768829000556, -3694.938000000000102, 2279.827800000000025 ) ) ;
#9772=ORIENTED_EDGE ( 'NONE', *, *, #9000, .T. ) ;
#9785=CARTESIAN_POINT ( 'NONE',  ( 22.54063073453000143, -3544.061999999999898, 2275.001800000000003 ) ) ;
#9791=DIRECTION ( 'NONE',  ( 0.000000000000000000, 0.000000000000000000, -1.000000000000000000 ) ) ;
#9793=EDGE_LOOP ( 'NONE', ( #7953, #6397, #1036, #9076 ) ) ;
#9795=ADVANCED_FACE ( 'NONE', ( #2147 ), #19726, .F. ) ;
#9820=DIRECTION ( 'NONE',  ( -1.000000000000000000, -1.935622821353000237E-14, 0.000000000000000000 ) ) ;
#9823=ORIENTED_EDGE ( 'NONE', *, *, #6105, .F. ) ;
#9832=ORIENTED_EDGE ( 'NONE', *, *, #2128, .T. ) ;
#9839=CARTESIAN_POINT ( 'NONE',  ( 9.855199999999999960, -3639.502500000000055, 2263.571799999999712 ) ) ;
#9861=EDGE_LOOP ( 'NONE', ( #11508, #6359 ) ) ;
#9874=CARTESIAN_POINT ( 'NONE',  ( 0.7620000000000000107, -3544.061999999999898, 2275.001800000000003 ) ) ;
#9879=VERTEX_POINT ( 'NONE', #20403 ) ;
#9884=FACE_OUTER_BOUND ( 'NONE', #18960, .T. ) ;
#9891=CARTESIAN_POINT ( 'NONE',  ( 64.76999999999999602, -3544.061999999999898, 2289.213099999999940 ) ) ;
#9897=DIRECTION ( 'NONE',  ( -1.000000000000000000, 0.000000000000000000, 0.000000000000000000 ) ) ;
#9900=ORIENTED_EDGE ( 'NONE', *, *, #19404, .T. ) ;
#9925=EDGE_LOOP ( 'NONE', ( #11674, #2854, #15695, #4889 ) ) ;
#9932=AXIS2_PLACEMENT_3D ( 'NONE', #16061, #21110, #5053 ) ;
#9935=EDGE_CURVE ( 'NONE', #8878, #9083, #22369, .T. ) ;
#9937=VERTEX_POINT ( 'NONE', #17691 ) ;
#9941=EDGE_CURVE ( 'NONE', #1484, #10742, #18268, .T. ) ;
#9947=CIRCLE ( 'NONE', #18192, 2.844799999999999773 ) ;
#9949=ORIENTED_EDGE ( 'NONE', *, *, #21970, .F. ) ;
#9950=CARTESIAN_POINT ( 'NONE',  ( 12.69999999999999929, -3639.502500000000055, 2295.829799999999977 ) ) ;
#9952=ORIENTED_EDGE ( 'NONE', *, *, #13454, .F. ) ;
#9957=AXIS2_PLACEMENT_3D ( 'NONE', #13790, #880, #6303 ) ;
#9960=DIRECTION ( 'NONE',  ( 0.000000000000000000, -1.000000000000000000, 0.000000000000000000 ) ) ;
#9972=DIRECTION ( 'NONE',  ( 0.000000000000000000, 0.000000000000000000, 1.000000000000000000 ) ) ;
#9981=EDGE_CURVE ( 'NONE', #2446, #20779, #3739, .T. ) ;
#9985=( LENGTH_UNIT ( ) NAMED_UNIT ( * ) SI_UNIT ( .MILLI., .METRE. ) );
#9995=EDGE_CURVE ( 'NONE', #22409, #1396, #14304, .T. ) ;
#10020=ORIENTED_EDGE ( 'NONE', *, *, #1, .T. ) ;
#10038=CARTESIAN_POINT ( 'NONE',  ( 20.32000000000000028, -3544.061999999999898, 2292.819899999999961 ) ) ;
#10045=ORIENTED_EDGE ( 'NONE', *, *, #18836, .T. ) ;
#10053=DIRECTION ( 'NONE',  ( 1.000000000000000000, -0.000000000000000000, 1.224646799147353207E-16 ) ) ;
#10059=VERTEX_POINT ( 'NONE', #10664 ) ;
#10087=DIRECTION ( 'NONE',  ( 1.000000000000000000, 0.000000000000000000, 0.000000000000000000 ) ) ;
#10094=FACE_OUTER_BOUND ( 'NONE', #20329, .T. ) ;
#10097=LINE ( 'NONE', #20123, #19943 ) ;
#10102=CARTESIAN_POINT ( 'NONE',  ( 9.209369265467998389, -3543.299999999999727, 2282.113800000000083 ) ) ;
#10104=LINE ( 'NONE', #1551, #20804 ) ;
#10112=CIRCLE ( 'NONE', #18350, 2.844799999999999773 ) ;
#10118=DIRECTION ( 'NONE',  ( 0.000000000000000000, 1.000000000000000000, 0.000000000000000000 ) ) ;
#10155=DIRECTION ( 'NONE',  ( 0.000000000000000000, 0.000000000000000000, -1.000000000000000000 ) ) ;
#10162=FACE_OUTER_BOUND ( 'NONE', #6177, .T. ) ;
#10166=ORIENTED_EDGE ( 'NONE', *, *, #19404, .F. ) ;
#10181=ORIENTED_EDGE ( 'NONE', *, *, #14636, .F. ) ;
#10209=CARTESIAN_POINT ( 'NONE',  ( 20.32000000000000028, -3568.700000000000273, 2289.213099999999940 ) ) ;
#10210=ORIENTED_EDGE ( 'NONE', *, *, #14723, .F. ) ;
#10212=DIRECTION ( 'NONE',  ( 0.000000000000000000, 0.000000000000000000, -1.000000000000000000 ) ) ;
#10228=ADVANCED_FACE ( 'NONE', ( #22706 ), #20841, .F. ) ;
#10231=ORIENTED_EDGE ( 'NONE', *, *, #20299, .F. ) ;
#10237=VERTEX_POINT ( 'NONE', #18968 ) ;
#10255=SPHERICAL_SURFACE ( 'NONE', #16081, 0.7620000000000000107 ) ;
#10268=CARTESIAN_POINT ( 'NONE',  ( 55.57575231171000496, -3695.699999999999818, 2275.763800000000174 ) ) ;
#10286=CIRCLE ( 'NONE', #22248, 5.714999999999999858 ) ;
#10298=LINE ( 'NONE', #1502, #9182 ) ;
#10327=VECTOR ( 'NONE', #9501, 1000.000000000000000 ) ;
#10339=AXIS2_PLACEMENT_3D ( 'NONE', #4976, #17270, #15645 ) ;
#10350=ORIENTED_EDGE ( 'NONE', *, *, #5216, .T. ) ;
#10354=ORIENTED_EDGE ( 'NONE', *, *, #16396, .T. ) ;
#10371=EDGE_CURVE ( 'NONE', #2446, #1205, #9947, .T. ) ;
#10383=DIRECTION ( 'NONE',  ( -1.000000000000000000, 0.000000000000000000, 0.000000000000000000 ) ) ;
#10399=ORIENTED_EDGE ( 'NONE', *, *, #12163, .T. ) ;
#10402=CARTESIAN_POINT ( 'NONE',  ( 20.32000000000000028, -3694.938000000000102, 2289.213099999999940 ) ) ;
#10409=ORIENTED_EDGE ( 'NONE', *, *, #18405, .T. ) ;
#10413=DIRECTION ( 'NONE',  ( -5.122214988120328377E-14, 0.000000000000000000, -1.000000000000000000 ) ) ;
#10435=ORIENTED_EDGE ( 'NONE', *, *, #7928, .F. ) ;
#10442=DIRECTION ( 'NONE',  ( 0.000000000000000000, 1.000000000000000000, 0.000000000000000000 ) ) ;
#10463=FACE_OUTER_BOUND ( 'NONE', #16514, .T. ) ;
#10465=ORIENTED_EDGE ( 'NONE', *, *, #13444, .T. ) ;
#10474=DIRECTION ( 'NONE',  ( 0.000000000000000000, 0.000000000000000000, -1.000000000000000000 ) ) ;
#10479=FACE_OUTER_BOUND ( 'NONE', #9793, .T. ) ;
#10529=( BOUNDED_CURVE ( )  B_SPLINE_CURVE ( 3, ( #7489, #21446, #12765, #1632 ),
 .UNSPECIFIED., .F., .T. ) 
 B_SPLINE_CURVE_WITH_KNOTS ( ( 4, 4 ),
 ( 3.141592653589793116, 4.712388980444761621 ),
 .UNSPECIFIED. ) 
 CURVE ( )  GEOMETRIC_REPRESENTATION_ITEM ( )  RATIONAL_B_SPLINE_CURVE ( ( 1.000000000000000000, 0.8047378541102059302, 0.8047378541102059302, 1.000000000000000000 ) ) 
 REPRESENTATION_ITEM ( '' )  );
#10534=AXIS2_PLACEMENT_3D ( 'NONE', #16371, #2200, #7466 ) ;
#10549=DIRECTION ( 'NONE',  ( 0.000000000000000000, 0.000000000000000000, -1.000000000000000000 ) ) ;
#10552=ADVANCED_FACE ( 'NONE', ( #3213 ), #17506, .T. ) ;
#10567=DIRECTION ( 'NONE',  ( 0.000000000000000000, 0.000000000000000000, -1.000000000000000000 ) ) ;
#10605=EDGE_CURVE ( 'NONE', #2058, #14578, #22302, .T. ) ;
#10607=AXIS2_PLACEMENT_3D ( 'NONE', #14552, #23084, #5646 ) ;
#10610=EDGE_LOOP ( 'NONE', ( #13109, #21749, #9614 ) ) ;
#10612=CARTESIAN_POINT ( 'NONE',  ( 19.17699999999999960, -3639.502500000000055, 2296.591799999999694 ) ) ;
#10639=VECTOR ( 'NONE', #11078, 1000.000000000000000 ) ;
#10647=EDGE_CURVE ( 'NONE', #6290, #2806, #4358, .T. ) ;
#10664=CARTESIAN_POINT ( 'NONE',  ( 61.26424768829000556, -3544.061999999999898, 2279.827800000000025 ) ) ;
#10674=CARTESIAN_POINT ( 'NONE',  ( 3.175000000260485677, -3695.384369265535042, 2275.001800000000003 ) ) ;
#10689=PRODUCT_CONTEXT ( 'NONE', #3350, 'mechanical' ) ;
#10693=EDGE_LOOP ( 'NONE', ( #20635, #4431, #3623, #10808 ) ) ;
#10696=VECTOR ( 'NONE', #7005, 1000.000000000000000 ) ;
#10726=ADVANCED_FACE ( 'NONE', ( #18320 ), #9424, .T. ) ;
#10741=AXIS2_PLACEMENT_3D ( 'NONE', #21173, #14373, #5701 ) ;
#10742=VERTEX_POINT ( 'NONE', #7091 ) ;
#10753=CARTESIAN_POINT ( 'NONE',  ( 22.54063073453000143, -3544.061999999999898, 2275.763800000000174 ) ) ;
#10761=ORIENTED_EDGE ( 'NONE', *, *, #16429, .T. ) ;
#10762=CARTESIAN_POINT ( 'NONE',  ( 0.000000000000000000, -3544.061999999999898, 2295.829799999999977 ) ) ;
#10766=CARTESIAN_POINT ( 'NONE',  ( 20.32000000000000028, -3544.061999999999898, 2289.213099999999940 ) ) ;
#10786=ORIENTED_EDGE ( 'NONE', *, *, #12962, .F. ) ;
#10792=PLANE ( 'NONE',  #14744 ) ;
#10794=ORIENTED_EDGE ( 'NONE', *, *, #21710, .F. ) ;
#10808=ORIENTED_EDGE ( 'NONE', *, *, #20587, .F. ) ;
#10815=EDGE_CURVE ( 'NONE', #11168, #8878, #5878, .T. ) ;
#10830=CARTESIAN_POINT ( 'NONE',  ( 61.26424768829000556, -3694.938000000000102, 2279.065800000000309 ) ) ;
#10840=CARTESIAN_POINT ( 'NONE',  ( 151.4000000000000057, -3694.938000000000102, 2280.589800000000196 ) ) ;
#10852=EDGE_LOOP ( 'NONE', ( #7328, #19958, #15072, #17321 ) ) ;
#10865=DIRECTION ( 'NONE',  ( 0.000000000000000000, -1.000000000000000000, 0.000000000000000000 ) ) ;
#10875=FACE_OUTER_BOUND ( 'NONE', #12559, .T. ) ;
#10909=CYLINDRICAL_SURFACE ( 'NONE', #10607, 2.844800000000091700 ) ;
#10910=ORIENTED_EDGE ( 'NONE', *, *, #21106, .F. ) ;
#10912=DIRECTION ( 'NONE',  ( 0.000000000000000000, -1.000000000000000000, 0.000000000000000000 ) ) ;
#10917=AXIS2_PLACEMENT_3D ( 'NONE', #1901, #12222, #5196 ) ;
#10923=DIRECTION ( 'NONE',  ( -5.122214988120328377E-14, 0.000000000000000000, -1.000000000000000000 ) ) ;
#10930=VERTEX_POINT ( 'NONE', #20604 ) ;
#10935=CARTESIAN_POINT ( 'NONE',  ( 12.69999999999999929, -3639.502500000000055, 2295.829799999999977 ) ) ;
#10939=CARTESIAN_POINT ( 'NONE',  ( 64.76999999999999602, -3695.699999999999818, 2285.606299999999919 ) ) ;
#10953=ORIENTED_EDGE ( 'NONE', *, *, #14605, .F. ) ;
#10967=ORIENTED_EDGE ( 'NONE', *, *, #15657, .F. ) ;
#10980=CYLINDRICAL_SURFACE ( 'NONE', #10534, 2.844800000000091700 ) ;
#10992=DIRECTION ( 'NONE',  ( 0.000000000000000000, 0.000000000000000000, 1.000000000000000000 ) ) ;
#11009=ADVANCED_FACE ( 'NONE', ( #7967 ), #20495, .F. ) ;
#11022=DIRECTION ( 'NONE',  ( 0.000000000000000000, 0.000000000000000000, -1.000000000000000000 ) ) ;
#11029=VERTEX_POINT ( 'NONE', #8775 ) ;
#11034=ORIENTED_EDGE ( 'NONE', *, *, #2416, .F. ) ;
#11043=AXIS2_PLACEMENT_3D ( 'NONE', #10209, #19355, #1423 ) ;
#11049=CIRCLE ( 'NONE', #17389, 0.7619999999999294005 ) ;
#11055=PLANE ( 'NONE',  #18756 ) ;
#11063=AXIS2_PLACEMENT_3D ( 'NONE', #20575, #5960, #2890 ) ;
#11066=CIRCLE ( 'NONE', #14069, 3.606800000000021100 ) ;
#11078=DIRECTION ( 'NONE',  ( 0.000000000000000000, 0.000000000000000000, 1.000000000000000000 ) ) ;
#11112=DIRECTION ( 'NONE',  ( 1.000000000000000000, 1.730170395987999916E-13, 0.000000000000000000 ) ) ;
#11115=DIRECTION ( 'NONE',  ( -1.000000000000000000, 0.000000000000000000, 0.000000000000000000 ) ) ;
#11124=CARTESIAN_POINT ( 'NONE',  ( 151.4000000000000057, -3543.299999999999727, 2275.001800000000003 ) ) ;
#11126=CIRCLE ( 'NONE', #10741, 6.477000000000000313 ) ;
#11134=CARTESIAN_POINT ( 'NONE',  ( 64.76999999999999602, -3694.938000000000102, 2289.213099999999940 ) ) ;
#11162=VERTEX_POINT ( 'NONE', #11936 ) ;
#11168=VERTEX_POINT ( 'NONE', #14633 ) ;
#11180=DIRECTION ( 'NONE',  ( -1.000000000000000000, -0.000000000000000000, -0.000000000000000000 ) ) ;
#11191=PLANE ( 'NONE',  #17381 ) ;
#11199=TOROIDAL_SURFACE ( 'NONE', #20934, 6.476999999999000224, 0.7620000000000000107 ) ;
#11206=ORIENTED_EDGE ( 'NONE', *, *, #4101, .T. ) ;
#11219=ORIENTED_EDGE ( 'NONE', *, *, #16954, .F. ) ;
#11235=DIRECTION ( 'NONE',  ( 1.000000000000000000, 0.000000000000000000, 1.344294159210000097E-14 ) ) ;
#11287=EDGE_CURVE ( 'NONE', #20662, #19560, #7702, .T. ) ;
#11297=CARTESIAN_POINT ( 'NONE',  ( 22.22500000000000142, -3543.299999999999727, 2275.001800000000003 ) ) ;
#11312=DIRECTION ( 'NONE',  ( 0.000000000000000000, 0.000000000000000000, -1.000000000000000000 ) ) ;
#11319=CARTESIAN_POINT ( 'NONE',  ( 61.26424768829000556, -3694.938000000000102, 2280.589800000000196 ) ) ;
#11333=ORIENTED_EDGE ( 'NONE', *, *, #20734, .F. ) ;
#11356=ADVANCED_FACE ( 'NONE', ( #2320 ), #5617, .F. ) ;
#11363=ADVANCED_FACE ( 'NONE', ( #13552 ), #21995, .T. ) ;
#11394=CYLINDRICAL_SURFACE ( 'NONE', #3548, 0.7619999999999231832 ) ;
#11408=ORIENTED_EDGE ( 'NONE', *, *, #12414, .F. ) ;
#11422=ADVANCED_FACE ( 'NONE', ( #6766 ), #15667, .F. ) ;
#11424=CIRCLE ( 'NONE', #7309, 2.844799999999999773 ) ;
#11503=AXIS2_PLACEMENT_3D ( 'NONE', #14389, #1734, #3709 ) ;
#11508=ORIENTED_EDGE ( 'NONE', *, *, #9724, .T. ) ;
#11516=EDGE_CURVE ( 'NONE', #10930, #16884, #22081, .T. ) ;
#11530=ORIENTED_EDGE ( 'NONE', *, *, #7106, .T. ) ;
#11544=DIRECTION ( 'NONE',  ( -0.7249994335945980639, 0.000000000000000000, -0.6887494619144990393 ) ) ;
#11546=FACE_OUTER_BOUND ( 'NONE', #3311, .T. ) ;
#11570=CARTESIAN_POINT ( 'NONE',  ( 20.32000000000000028, -3694.938000000000102, 2292.057900000000245 ) ) ;
#11576=EDGE_CURVE ( 'NONE', #4104, #20566, #7662, .T. ) ;
#11579=DIRECTION ( 'NONE',  ( 0.000000000000000000, 0.000000000000000000, 1.000000000000000000 ) ) ;
#11625=CARTESIAN_POINT ( 'NONE',  ( 0.000000000000000000, -3694.938000000000102, 2295.829799999999977 ) ) ;
#11648=ORIENTED_EDGE ( 'NONE', *, *, #8263, .F. ) ;
#11652=CARTESIAN_POINT ( 'NONE',  ( 12.69999999999999929, -3639.502500000000055, 2281.351799999999912 ) ) ;
#11657=DIRECTION ( 'NONE',  ( 0.000000000000000000, -1.000000000000000000, 0.000000000000000000 ) ) ;
#11667=CIRCLE ( 'NONE', #20653, 2.844800000000091700 ) ;
#11674=ORIENTED_EDGE ( 'NONE', *, *, #3981, .T. ) ;
#11682=AXIS2_PLACEMENT_3D ( 'NONE', #12574, #17957, #8943 ) ;
#11709=DIRECTION ( 'NONE',  ( 1.000000000000000000, 0.000000000000000000, 2.117363008798000070E-13 ) ) ;
#11736=VECTOR ( 'NONE', #21548, 1000.000000000000000 ) ;
#11742=LINE ( 'NONE', #22518, #2831 ) ;
#11745=CYLINDRICAL_SURFACE ( 'NONE', #18634, 0.7619999999999294005 ) ;
#11760=ORIENTED_EDGE ( 'NONE', *, *, #15973, .T. ) ;
#11766=DIRECTION ( 'NONE',  ( 0.000000000000000000, -1.000000000000000000, 0.000000000000000000 ) ) ;
#11776=EDGE_CURVE ( 'NONE', #4616, #3230, #14917, .T. ) ;
#11777=CARTESIAN_POINT ( 'NONE',  ( 16.00573853068664931, -3543.299999999971988, 2281.667430734553363 ) ) ;
#11783=CIRCLE ( 'NONE', #2449, 2.844799999999999773 ) ;
#11790=CIRCLE ( 'NONE', #1696, 2.844800000000091700 ) ;
#11792=AXIS2_PLACEMENT_3D ( 'NONE', #8350, #19359, #15491 ) ;
#11821=ORIENTED_EDGE ( 'NONE', *, *, #8516, .T. ) ;
#11823=VECTOR ( 'NONE', #15518, 1000.000000000000000 ) ;
#11832=ADVANCED_FACE ( 'NONE', ( #13020 ), #20375, .T. ) ;
#11834=VERTEX_POINT ( 'NONE', #3749 ) ;
#11835=CARTESIAN_POINT ( 'NONE',  ( 64.76999999999999602, -3568.700000000000273, 2286.368300000000090 ) ) ;
#11850=ADVANCED_FACE ( 'NONE', ( #5765 ), #3874, .T. ) ;
#11863=VECTOR ( 'NONE', #8477, 1000.000000000000000 ) ;
#11876=CARTESIAN_POINT ( 'NONE',  ( 20.32000000000000028, -3670.300000000000182, 2286.368300000000090 ) ) ;
#11887=ORIENTED_EDGE ( 'NONE', *, *, #12666, .T. ) ;
#11920=FACE_OUTER_BOUND ( 'NONE', #5127, .T. ) ;
#11925=CARTESIAN_POINT ( 'NONE',  ( 12.69999999999999929, -3639.502500000000055, 2295.829799999999977 ) ) ;
#11936=CARTESIAN_POINT ( 'NONE',  ( 20.32000000000000028, -3568.700000000000273, 2292.057900000000245 ) ) ;
#11949=ADVANCED_FACE ( 'NONE', ( #7970 ), #8197, .F. ) ;
#11950=CARTESIAN_POINT ( 'NONE',  ( 6.222999999999998977, -3639.502500000000055, 2295.829799999999977 ) ) ;
#11989=ORIENTED_EDGE ( 'NONE', *, *, #12962, .T. ) ;
#12034=DIRECTION ( 'NONE',  ( 0.000000000000000000, 1.000000000000000000, 0.000000000000000000 ) ) ;
#12036=DIRECTION ( 'NONE',  ( 0.000000000000000000, -1.000000000000000000, 0.000000000000000000 ) ) ;
#12038=AXIS2_PLACEMENT_3D ( 'NONE', #15157, #7785, #21849 ) ;
#12039=ORIENTED_EDGE ( 'NONE', *, *, #15026, .F. ) ;
#12064=DIRECTION ( 'NONE',  ( -0.000000000000000000, -1.000000000000000000, -0.000000000000000000 ) ) ;
#12076=EDGE_CURVE ( 'NONE', #4616, #6734, #18731, .T. ) ;
#12081=ORIENTED_EDGE ( 'NONE', *, *, #21106, .T. ) ;
#12083=VERTEX_POINT ( 'NONE', #16861 ) ;
#12102=DIRECTION ( 'NONE',  ( -1.000000000000000000, 0.000000000000000000, 0.000000000000000000 ) ) ;
#12107=ORIENTED_EDGE ( 'NONE', *, *, #7962, .F. ) ;
#12115=VERTEX_POINT ( 'NONE', #21086 ) ;
#12116=CYLINDRICAL_SURFACE ( 'NONE', #2294, 0.7619999999999230722 ) ;
#12137=DIRECTION ( 'NONE',  ( 0.000000000000000000, 0.000000000000000000, -1.000000000000000000 ) ) ;
#12148=VECTOR ( 'NONE', #20469, 1000.000000000000000 ) ;
#12163=EDGE_CURVE ( 'NONE', #5531, #5311, #14056, .T. ) ;
#12171=AXIS2_PLACEMENT_3D ( 'NONE', #21120, #10212, #6829 ) ;
#12184=PLANE ( 'NONE',  #20083 ) ;
#12198=VECTOR ( 'NONE', #20143, 1000.000000000000000 ) ;
#12202=FACE_OUTER_BOUND ( 'NONE', #3895, .T. ) ;
#12214=EDGE_CURVE ( 'NONE', #2445, #11162, #11790, .T. ) ;
#12221=CARTESIAN_POINT ( 'NONE',  ( 61.26424768829000556, -3543.299999999999727, 2279.065800000000309 ) ) ;
#12222=DIRECTION ( 'NONE',  ( 1.000000000000000000, 0.000000000000000000, 0.000000000000000000 ) ) ;
#12234=AXIS2_PLACEMENT_3D ( 'NONE', #1930, #16223, #4036 ) ;
#12251=ORIENTED_EDGE ( 'NONE', *, *, #18022, .T. ) ;
#12254=ORIENTED_EDGE ( 'NONE', *, *, #22504, .F. ) ;
#12260=EDGE_LOOP ( 'NONE', ( #4528, #14465, #21759, #6067 ) ) ;
#12284=EDGE_CURVE ( 'NONE', #5265, #8260, #10298, .T. ) ;
#12308=ORIENTED_EDGE ( 'NONE', *, *, #12284, .T. ) ;
#12323=DIRECTION ( 'NONE',  ( -0.7071067811865969777, 0.000000000000000000, -0.7071067811864980568 ) ) ;
#12326=ORIENTED_EDGE ( 'NONE', *, *, #22514, .T. ) ;
#12327=DIRECTION ( 'NONE',  ( 0.000000000000000000, -1.000000000000000000, 0.000000000000000000 ) ) ;
#12334=FACE_OUTER_BOUND ( 'NONE', #6639, .T. ) ;
#12339=FACE_OUTER_BOUND ( 'NONE', #6496, .T. ) ;
#12342=CARTESIAN_POINT ( 'NONE',  ( 0.7620000000000000107, -3544.061999999999898, 2275.763800000000174 ) ) ;
#12347=DIRECTION ( 'NONE',  ( 0.000000000000000000, 1.000000000000000000, 0.000000000000000000 ) ) ;
#12353=CARTESIAN_POINT ( 'NONE',  ( 22.54063073453000143, -3694.938000000000102, 2275.763800000000174 ) ) ;
#12379=DIRECTION ( 'NONE',  ( -1.000000000000000000, 0.000000000000000000, 0.000000000000000000 ) ) ;
#12398=DIRECTION ( 'NONE',  ( 0.000000000000000000, 0.000000000000000000, 1.000000000000000000 ) ) ;
#12400=VERTEX_POINT ( 'NONE', #16158 ) ;
#12414=EDGE_CURVE ( 'NONE', #5647, #7405, #19909, .T. ) ;
#12425=DIRECTION ( 'NONE',  ( 1.000000000000000000, 0.000000000000000000, 0.000000000000000000 ) ) ;
#12432=FACE_OUTER_BOUND ( 'NONE', #9514, .T. ) ;
#12443=AXIS2_PLACEMENT_3D ( 'NONE', #21931, #15796, #3019 ) ;
#12444=ORIENTED_EDGE ( 'NONE', *, *, #11287, .T. ) ;
#12452=PLANE ( 'NONE',  #10917 ) ;
#12459=VERTEX_POINT ( 'NONE', #20360 ) ;
#12465=ORIENTED_EDGE ( 'NONE', *, *, #2929, .T. ) ;
#12477=VECTOR ( 'NONE', #18892, 1000.000000000000000 ) ;
#12487=CIRCLE ( 'NONE', #6894, 2.844800000000091700 ) ;
#12499=CARTESIAN_POINT ( 'NONE',  ( 18.41499999999899728, -3599.497499999999945, 2288.971800000000258 ) ) ;
#12505=EDGE_CURVE ( 'NONE', #6730, #5647, #20826, .T. ) ;
#12511=CARTESIAN_POINT ( 'NONE',  ( 60.21459350834000190, -3694.938000000000102, 2280.170699136999701 ) ) ;
#12546=EDGE_LOOP ( 'NONE', ( #18633, #22895, #14485 ) ) ;
#12553=VECTOR ( 'NONE', #22935, 1000.000000000000114 ) ;
#12555=AXIS2_PLACEMENT_3D ( 'NONE', #15962, #3415, #10567 ) ;
#12559=EDGE_LOOP ( 'NONE', ( #10761, #7474, #20526, #9823 ) ) ;
#12574=CARTESIAN_POINT ( 'NONE',  ( 0.7620000000000000107, -3694.938000000000102, 2275.001800000000003 ) ) ;
#12577=AXIS2_PLACEMENT_3D ( 'NONE', #14285, #21431, #3721 ) ;
#12579=AXIS2_PLACEMENT_3D ( 'NONE', #19351, #358, #22210 ) ;
#12598=DIRECTION ( 'NONE',  ( -0.000000000000000000, 1.000000000000000000, 0.000000000000000000 ) ) ;
#12601=VECTOR ( 'NONE', #20686, 1000.000000000000000 ) ;
#12612=CARTESIAN_POINT ( 'NONE',  ( 15.54479999999999862, -3599.497499999999945, 2263.571799999999712 ) ) ;
#12632=DIRECTION ( 'NONE',  ( 0.7249994335957196112, -1.571266676791983932E-13, 0.6887494619133185392 ) ) ;
#12634=CARTESIAN_POINT ( 'NONE',  ( 3.175000000094025054, -3694.938000000000102, 2275.001800000090952 ) ) ;
#12666=EDGE_CURVE ( 'NONE', #9312, #3779, #14027, .T. ) ;
#12669=CARTESIAN_POINT ( 'NONE',  ( 20.32000000000000028, -3670.300000000000182, 2289.213099999999940 ) ) ;
#12713=EDGE_LOOP ( 'NONE', ( #3648, #6568, #10409, #5786 ) ) ;
#12716=LINE ( 'NONE', #14826, #2536 ) ;
#12722=CIRCLE ( 'NONE', #22420, 0.7619999999999294005 ) ;
#12737=CIRCLE ( 'NONE', #389, 0.7619999999999294005 ) ;
#12765=CARTESIAN_POINT ( 'NONE',  ( 9.394261469307407353, -3695.700000000027103, 2281.667430734552454 ) ) ;
#12773=EDGE_LOOP ( 'NONE', ( #7334, #13257, #2403, #6425 ) ) ;
#12777=EDGE_LOOP ( 'NONE', ( #7718, #18538, #3744, #21435 ) ) ;
#12778=LINE ( 'NONE', #3872, #14799 ) ;
#12779=ORIENTED_EDGE ( 'NONE', *, *, #9315, .T. ) ;
#12788=FACE_BOUND ( 'NONE', #16394, .T. ) ;
#12798=ORIENTED_EDGE ( 'NONE', *, *, #22900, .F. ) ;
#12812=CARTESIAN_POINT ( 'NONE',  ( 9.855199999999999960, -3599.497499999999945, 2288.971800000000258 ) ) ;
#12814=ORIENTED_EDGE ( 'NONE', *, *, #8238, .T. ) ;
#12819=CARTESIAN_POINT ( 'NONE',  ( 12.69999999999999929, -3639.502500000000055, 2296.591799999999694 ) ) ;
#12830=TOROIDAL_SURFACE ( 'NONE', #13952, 3.606799999999999784, 0.7620000000000000107 ) ;
#12856=AXIS2_PLACEMENT_3D ( 'NONE', #8547, #15690, #18845 ) ;
#12862=CARTESIAN_POINT ( 'NONE',  ( 0.7620000000000000107, -3544.061999999999898, 2295.829799999999977 ) ) ;
#12930=ADVANCED_FACE ( 'NONE', ( #16701 ), #20549, .F. ) ;
#12942=AXIS2_PLACEMENT_3D ( 'NONE', #4582, #9972, #948 ) ;
#12962=EDGE_CURVE ( 'NONE', #13565, #18622, #18504, .T. ) ;
#12970=CARTESIAN_POINT ( 'NONE',  ( 6.985000000000999520, -3599.497499999999945, 2295.829799999999977 ) ) ;
#12982=DIRECTION ( 'NONE',  ( 0.000000000000000000, 0.000000000000000000, 1.000000000000000000 ) ) ;
#12985=DIRECTION ( 'NONE',  ( 1.000000000000000000, 0.000000000000000000, 0.000000000000000000 ) ) ;
#12994=ORIENTED_EDGE ( 'NONE', *, *, #22441, .F. ) ;
#13020=FACE_OUTER_BOUND ( 'NONE', #1687, .T. ) ;
#13042=EDGE_CURVE ( 'NONE', #22793, #3779, #3922, .T. ) ;
#13054=LINE ( 'NONE', #20203, #1609 ) ;
#13081=CIRCLE ( 'NONE', #22042, 3.606800000000021100 ) ;
#13096=ORIENTED_EDGE ( 'NONE', *, *, #2824, .T. ) ;
#13109=ORIENTED_EDGE ( 'NONE', *, *, #2541, .T. ) ;
#13114=CIRCLE ( 'NONE', #15359, 2.844800000000091700 ) ;
#13124=DIRECTION ( 'NONE',  ( -1.000000000000000000, 0.000000000000000000, 0.000000000000000000 ) ) ;
#13128=CARTESIAN_POINT ( 'NONE',  ( 0.7620000000000000107, -3544.061999999999898, 2275.001800000000003 ) ) ;
#13129=ORIENTED_EDGE ( 'NONE', *, *, #22996, .F. ) ;
#13130=DIRECTION ( 'NONE',  ( -1.000000000000000000, 0.000000000000000000, 0.000000000000000000 ) ) ;
#13157=CIRCLE ( 'NONE', #3048, 2.844800000000091700 ) ;
#13181=VECTOR ( 'NONE', #18810, 1000.000000000000000 ) ;
#13222=FACE_OUTER_BOUND ( 'NONE', #18328, .T. ) ;
#13226=LINE ( 'NONE', #18972, #13247 ) ;
#13233=ORIENTED_EDGE ( 'NONE', *, *, #2541, .F. ) ;
#13236=ORIENTED_EDGE ( 'NONE', *, *, #5455, .F. ) ;
#13247=VECTOR ( 'NONE', #20377, 1000.000000000000000 ) ;
#13257=ORIENTED_EDGE ( 'NONE', *, *, #17070, .F. ) ;
#13263=VERTEX_POINT ( 'NONE', #10939 ) ;
#13277=AXIS2_PLACEMENT_3D ( 'NONE', #16123, #14491, #21858 ) ;
#13282=EDGE_CURVE ( 'NONE', #22793, #6119, #53, .T. ) ;
#13285=MANIFOLD_SOLID_BREP ( 'SOLID45-11[1]', #16962 ) ;
#13294=DIRECTION ( 'NONE',  ( 0.000000000000000000, 1.000000000000000000, 0.000000000000000000 ) ) ;
#13295=AXIS2_PLACEMENT_3D ( 'NONE', #15145, #2711, #22272 ) ;
#13309=VERTEX_POINT ( 'NONE', #3675 ) ;
#13313=AXIS2_PLACEMENT_3D ( 'NONE', #1724, #8872, #5828 ) ;
#13335=ORIENTED_EDGE ( 'NONE', *, *, #21976, .F. ) ;
#13340=CARTESIAN_POINT ( 'NONE',  ( 64.76999999999999602, -3695.699999999999818, 2289.213099999999940 ) ) ;
#13343=CARTESIAN_POINT ( 'NONE',  ( 20.32000000000000028, -3670.300000000000182, 2289.213099999999940 ) ) ;
#13363=CARTESIAN_POINT ( 'NONE',  ( 6.222999999999998977, -3639.502500000000055, 2296.591799999999694 ) ) ;
#13379=ORIENTED_EDGE ( 'NONE', *, *, #4508, .F. ) ;
#13383=ORIENTED_EDGE ( 'NONE', *, *, #18262, .F. ) ;
#13391=ADVANCED_FACE ( 'NONE', ( #841 ), #11394, .T. ) ;
#13412=VERTEX_POINT ( 'NONE', #510 ) ;
#13429=PLANE ( 'NONE',  #3525 ) ;
#13432=CIRCLE ( 'NONE', #5975, 5.714999999998998881 ) ;
#13439=CARTESIAN_POINT ( 'NONE',  ( 22.00181536726000076, -3544.061999999999898, 2275.224984633000076 ) ) ;
#13444=EDGE_CURVE ( 'NONE', #10237, #10059, #11049, .T. ) ;
#13454=EDGE_CURVE ( 'NONE', #6119, #20566, #2602, .T. ) ;
#13459=DIRECTION ( 'NONE',  ( 1.000000000000000000, 0.000000000000000000, 0.000000000000000000 ) ) ;
#13460=ORIENTED_EDGE ( 'NONE', *, *, #16700, .F. ) ;
#13461=AXIS2_PLACEMENT_3D ( 'NONE', #8793, #23072, #1519 ) ;
#13473=LINE ( 'NONE', #9839, #2152 ) ;
#13485=ORIENTED_EDGE ( 'NONE', *, *, #13936, .T. ) ;
#13494=DIRECTION ( 'NONE',  ( -0.7071067811865975328, 0.000000000000000000, -0.7071067811864976127 ) ) ;
#13497=AXIS2_PLACEMENT_3D ( 'NONE', #5363, #5134, #1729 ) ;
#13543=CARTESIAN_POINT ( 'NONE',  ( 15.87499999973273823, -3543.615630734505885, 2281.351799999999912 ) ) ;
#13546=ADVANCED_FACE ( 'NONE', ( #8470 ), #8812, .T. ) ;
#13547=DIRECTION ( 'NONE',  ( 0.000000000000000000, -1.000000000000000000, 0.000000000000000000 ) ) ;
#13551=AXIS2_PLACEMENT_3D ( 'NONE', #12511, #12632, #5496 ) ;
#13552=FACE_OUTER_BOUND ( 'NONE', #3755, .T. ) ;
#13557=DIRECTION ( 'NONE',  ( -0.7071067811865975328, 0.000000000000000000, 0.7071067811864976127 ) ) ;
#13565=VERTEX_POINT ( 'NONE', #6947 ) ;
#13576=ADVANCED_FACE ( 'NONE', ( #1071 ), #13853, .F. ) ;
#13578=AXIS2_PLACEMENT_3D ( 'NONE', #6773, #13913, #21065 ) ;
#13632=TOROIDAL_SURFACE ( 'NONE', #6538, 3.606799999999999784, 0.7620000000000000107 ) ;
#13635=ADVANCED_FACE ( 'NONE', ( #10094 ), #3647, .F. ) ;
#13642=EDGE_LOOP ( 'NONE', ( #5953, #12994, #6589, #3339 ) ) ;
#13645=CYLINDRICAL_SURFACE ( 'NONE', #21190, 0.7619999999999241824 ) ;
#13657=ORIENTED_EDGE ( 'NONE', *, *, #11776, .F. ) ;
#13672=ADVANCED_FACE ( 'NONE', ( #1888 ), #19940, .T. ) ;
#13692=ORIENTED_EDGE ( 'NONE', *, *, #19599, .T. ) ;
#13697=DIRECTION ( 'NONE',  ( 0.000000000000000000, 0.000000000000000000, -1.000000000000000000 ) ) ;
#13698=VECTOR ( 'NONE', #11709, 1000.000000000000000 ) ;
#13700=ORIENTED_EDGE ( 'NONE', *, *, #15602, .F. ) ;
#13733=AXIS2_PLACEMENT_3D ( 'NONE', #7338, #21635, #16575 ) ;
#13757=ADVANCED_FACE ( 'NONE', ( #21468 ), #4687, .T. ) ;
#13778=CARTESIAN_POINT ( 'NONE',  ( 9.525000000091798924, -3694.938000000000102, 2281.351800000090861 ) ) ;
#13783=CARTESIAN_POINT ( 'NONE',  ( 12.69999999999999929, -3599.497499999999945, 2296.591799999999694 ) ) ;
#13785=ORIENTED_EDGE ( 'NONE', *, *, #20587, .T. ) ;
#13790=CARTESIAN_POINT ( 'NONE',  ( 64.76999999999999602, -3694.938000000000102, 2285.606299999999919 ) ) ;
#13795=DIRECTION ( 'NONE',  ( -1.000000000000000000, 0.000000000000000000, 0.000000000000000000 ) ) ;
#13807=EDGE_CURVE ( 'NONE', #16242, #2028, #11424, .T. ) ;
#13811=EDGE_CURVE ( 'NONE', #22211, #9308, #14438, .T. ) ;
#13819=LINE ( 'NONE', #5150, #16611 ) ;
#13844=EDGE_LOOP ( 'NONE', ( #19310, #18053, #12081, #19639 ) ) ;
#13845=CIRCLE ( 'NONE', #363, 0.7619999999999294005 ) ;
#13853=PLANE ( 'NONE',  #11792 ) ;
#13879=ORIENTED_EDGE ( 'NONE', *, *, #22811, .F. ) ;
#13884=EDGE_LOOP ( 'NONE', ( #10045, #16916, #22106, #7434 ) ) ;
#13913=DIRECTION ( 'NONE',  ( 0.000000000000000000, -1.000000000000000000, 0.000000000000000000 ) ) ;
#13936=EDGE_CURVE ( 'NONE', #6119, #15991, #21809, .T. ) ;
#13937=CARTESIAN_POINT ( 'NONE',  ( 15.87500000000000000, -3694.938000000000102, 2281.351799999999912 ) ) ;
#13946=FACE_BOUND ( 'NONE', #1558, .T. ) ;
#13952=AXIS2_PLACEMENT_3D ( 'NONE', #5301, #20891, #1306 ) ;
#13978=CIRCLE ( 'NONE', #3868, 0.7619999999999294005 ) ;
#14004=ORIENTED_EDGE ( 'NONE', *, *, #16436, .F. ) ;
#14008=DIRECTION ( 'NONE',  ( 0.000000000000000000, 1.000000000000000000, 0.000000000000000000 ) ) ;
#14016=CARTESIAN_POINT ( 'NONE',  ( 0.7620000000000000107, -3544.061999999999898, 2295.829799999999977 ) ) ;
#14026=ORIENTED_EDGE ( 'NONE', *, *, #13936, .F. ) ;
#14027=LINE ( 'NONE', #10268, #2034 ) ;
#14056=LINE ( 'NONE', #17441, #21904 ) ;
#14069=AXIS2_PLACEMENT_3D ( 'NONE', #253, #18699, #2649 ) ;
#14077=ORIENTED_EDGE ( 'NONE', *, *, #4542, .F. ) ;
#14081=EDGE_LOOP ( 'NONE', ( #5566, #19535, #7304 ) ) ;
#14087=CIRCLE ( 'NONE', #9957, 0.7619999999999294005 ) ;
#14107=LINE ( 'NONE', #5315, #1358 ) ;
#14108=VERTEX_POINT ( 'NONE', #19043 ) ;
#14114=CARTESIAN_POINT ( 'NONE',  ( 18.41499999999899728, -3599.497499999999945, 2288.971800000000258 ) ) ;
#14145=CARTESIAN_POINT ( 'NONE',  ( 6.985000000000000320, -3639.502500000000055, 2295.829799999999977 ) ) ;
#14165=DIRECTION ( 'NONE',  ( 0.000000000000000000, 1.000000000000000000, 0.000000000000000000 ) ) ;
#14166=CARTESIAN_POINT ( 'NONE',  ( 20.32000000000000028, -3544.061999999999898, 2285.606299999999919 ) ) ;
#14170=ADVANCED_FACE ( 'NONE', ( #4286 ), #6984, .T. ) ;
#14186=ADVANCED_FACE ( 'NONE', ( #10479 ), #15877, .F. ) ;
#14195=CARTESIAN_POINT ( 'NONE',  ( 3.175000000091532382, -3544.061999999999898, 2275.001800000095045 ) ) ;
#14200=CARTESIAN_POINT ( 'NONE',  ( 20.32000000000000028, -3568.700000000000273, 2286.368300000000090 ) ) ;
#14206=PLANE ( 'NONE',  #8295 ) ;
#14221=CARTESIAN_POINT ( 'NONE',  ( 3.175000000091532382, -3544.061999999999898, 2275.001800000095045 ) ) ;
#14244=ORIENTED_EDGE ( 'NONE', *, *, #20973, .T. ) ;
#14247=AXIS2_PLACEMENT_3D ( 'NONE', #15916, #23048, #5373 ) ;
#14257=CYLINDRICAL_SURFACE ( 'NONE', #21232, 0.7619999999999294005 ) ;
#14261=ORIENTED_EDGE ( 'NONE', *, *, #4432, .F. ) ;
#14280=DIRECTION ( 'NONE',  ( 0.000000000000000000, 0.000000000000000000, 1.000000000000000000 ) ) ;
#14285=CARTESIAN_POINT ( 'NONE',  ( 12.69999999999999929, -3639.502500000000055, 2288.971800000000258 ) ) ;
#14291=ORIENTED_EDGE ( 'NONE', *, *, #2776, .F. ) ;
#14304=LINE ( 'NONE', #5633, #8879 ) ;
#14320=CYLINDRICAL_SURFACE ( 'NONE', #3933, 0.7619999999999294005 ) ;
#14323=TOROIDAL_SURFACE ( 'NONE', #16189, 6.477000000000000313, 0.7620000000000000107 ) ;
#14329=EDGE_CURVE ( 'NONE', #3812, #18833, #22562, .T. ) ;
#14347=EDGE_LOOP ( 'NONE', ( #6417, #6972 ) ) ;
#14353=AXIS2_PLACEMENT_3D ( 'NONE', #11134, #9486, #18619 ) ;
#14357=CARTESIAN_POINT ( 'NONE',  ( 152.4000000000000057, -3695.699999999999818, 2275.001800000000003 ) ) ;
#14373=DIRECTION ( 'NONE',  ( 0.000000000000000000, 0.000000000000000000, -1.000000000000000000 ) ) ;
#14383=ORIENTED_EDGE ( 'NONE', *, *, #14723, .T. ) ;
#14389=CARTESIAN_POINT ( 'NONE',  ( 64.76999999999999602, -3670.300000000000182, 2289.213099999999940 ) ) ;
#14401=AXIS2_PLACEMENT_3D ( 'NONE', #5821, #8867, #7111 ) ;
#14414=ORIENTED_EDGE ( 'NONE', *, *, #15229, .F. ) ;
#14438=CIRCLE ( 'NONE', #4309, 2.844800000000091700 ) ;
#14443=ORIENTED_EDGE ( 'NONE', *, *, #18377, .F. ) ;
#14452=EDGE_LOOP ( 'NONE', ( #10020, #8661, #22223 ) ) ;
#14465=ORIENTED_EDGE ( 'NONE', *, *, #16446, .T. ) ;
#14474=DIRECTION ( 'NONE',  ( 1.000000000000000000, 0.000000000000000000, 0.000000000000000000 ) ) ;
#14485=ORIENTED_EDGE ( 'NONE', *, *, #22461, .T. ) ;
#14486=CARTESIAN_POINT ( 'NONE',  ( 16.19063073443439293, -3695.699999999999818, 2282.113800000095125 ) ) ;
#14487=DIRECTION ( 'NONE',  ( 0.000000000000000000, 0.000000000000000000, -1.000000000000000000 ) ) ;
#14491=DIRECTION ( 'NONE',  ( 0.000000000000000000, 1.000000000000000000, 0.000000000000000000 ) ) ;
#14495=CARTESIAN_POINT ( 'NONE',  ( 15.87499999973130826, -3695.384369265537771, 2281.351799999999912 ) ) ;
#14508=AXIS2_PLACEMENT_3D ( 'NONE', #7629, #22259, #2697 ) ;
#14518=DIRECTION ( 'NONE',  ( 0.000000000000000000, 0.000000000000000000, -1.000000000000000000 ) ) ;
#14524=ORIENTED_EDGE ( 'NONE', *, *, #19599, .F. ) ;
#14552=CARTESIAN_POINT ( 'NONE',  ( 64.76999999999999602, -3670.300000000000182, 2289.213099999999940 ) ) ;
#14571=EDGE_CURVE ( 'NONE', #11834, #10742, #16672, .T. ) ;
#14578=VERTEX_POINT ( 'NONE', #9752 ) ;
#14580=CARTESIAN_POINT ( 'NONE',  ( 64.76999999999999602, -3670.300000000000182, 2289.213099999999940 ) ) ;
#14600=TOROIDAL_SURFACE ( 'NONE', #1109, 3.606799999999999784, 0.7620000000000000107 ) ;
#14602=CARTESIAN_POINT ( 'NONE',  ( 60.73942059830999796, -3544.061999999999898, 2279.618249568000010 ) ) ;
#14605=EDGE_CURVE ( 'NONE', #9312, #22767, #13054, .T. ) ;
#14631=CARTESIAN_POINT ( 'NONE',  ( 56.10057940169000545, -3694.938000000000102, 2275.211350432000472 ) ) ;
#14633=CARTESIAN_POINT ( 'NONE',  ( 18.41499999999899728, -3599.497499999999945, 2295.829799999999977 ) ) ;
#14636=EDGE_CURVE ( 'NONE', #1414, #20799, #2169, .T. ) ;
#14694=DIRECTION ( 'NONE',  ( 0.000000000000000000, 0.000000000000000000, -1.000000000000000000 ) ) ;
#14711=FACE_OUTER_BOUND ( 'NONE', #21442, .T. ) ;
#14720=CARTESIAN_POINT ( 'NONE',  ( 16.00573853070648767, -3695.700000000083946, 2281.667430734605205 ) ) ;
#14723=EDGE_CURVE ( 'NONE', #4922, #6249, #3454, .T. ) ;
#14744=AXIS2_PLACEMENT_3D ( 'NONE', #8921, #7168, #21804 ) ;
#14746=DIRECTION ( 'NONE',  ( 0.000000000000000000, -1.000000000000000000, 0.000000000000000000 ) ) ;
#14750=CARTESIAN_POINT ( 'NONE',  ( 60.73942059830999796, -3694.938000000000102, 2279.618249568000010 ) ) ;
#14775=CARTESIAN_POINT ( 'NONE',  ( 0.000000000000000000, -3544.061999999999898, 2280.589800000000196 ) ) ;
#14799=VECTOR ( 'NONE', #9385, 1000.000000000000000 ) ;
#14802=AXIS2_PLACEMENT_3D ( 'NONE', #16190, #9160, #142 ) ;
#14803=EDGE_LOOP ( 'NONE', ( #8146, #19491, #19951, #16165 ) ) ;
#14804=DIRECTION ( 'NONE',  ( 0.000000000000000000, 1.000000000000000000, 0.000000000000000000 ) ) ;
#14826=CARTESIAN_POINT ( 'NONE',  ( 0.000000000000000000, -3544.061999999999898, 2275.763800000000174 ) ) ;
#14844=CARTESIAN_POINT ( 'NONE',  ( 9.525000000092171959, -3544.061999999999898, 2281.351800000095409 ) ) ;
#14863=EDGE_LOOP ( 'NONE', ( #17027, #2925 ) ) ;
#14882=ADVANCED_FACE ( 'NONE', ( #17681 ), #17453, .T. ) ;
#14900=EDGE_CURVE ( 'NONE', #15991, #9312, #20651, .T. ) ;
#14917=( BOUNDED_CURVE ( )  B_SPLINE_CURVE ( 3, ( #15401, #10674, #3086, #1088 ),
 .UNSPECIFIED., .F., .T. ) 
 B_SPLINE_CURVE_WITH_KNOTS ( ( 4, 4 ),
 ( 0.000000000000000000, 1.570796326975000712 ),
 .UNSPECIFIED. ) 
 CURVE ( )  GEOMETRIC_REPRESENTATION_ITEM ( )  RATIONAL_B_SPLINE_CURVE ( ( 1.000000000000000000, 0.8047378540819140058, 0.8047378540819140058, 1.000000000000000000 ) ) 
 REPRESENTATION_ITEM ( '' )  );
#14923=EDGE_LOOP ( 'NONE', ( #8089, #18466, #3658, #4509 ) ) ;
#14924=CARTESIAN_POINT ( 'NONE',  ( 9.524999999998000177, -3694.938000000000102, 2281.351799999999912 ) ) ;
#14935=DIRECTION ( 'NONE',  ( -0.7071067811866180719, 0.000000000000000000, -0.7071067811864769626 ) ) ;
#14947=EDGE_LOOP ( 'NONE', ( #13096, #4627, #7402, #21302 ) ) ;
#14951=CIRCLE ( 'NONE', #4833, 0.7619999999999294005 ) ;
#14952=FACE_OUTER_BOUND ( 'NONE', #3435, .T. ) ;
#14953=CARTESIAN_POINT ( 'NONE',  ( 60.21459350834000190, -3695.699999999999818, 2280.170699136999701 ) ) ;
#14960=DIRECTION ( 'NONE',  ( 0.000000000000000000, 0.000000000000000000, -1.000000000000000000 ) ) ;
#14966=DIRECTION ( 'NONE',  ( -0.7249994335945011414, -3.300980413455180170E-14, -0.6887494619146010688 ) ) ;
#14987=ORIENTED_EDGE ( 'NONE', *, *, #20010, .T. ) ;
#15003=CARTESIAN_POINT ( 'NONE',  ( 3.175000000003000089, -3694.938000000000102, 2275.001800000000003 ) ) ;
#15006=EDGE_LOOP ( 'NONE', ( #15261, #1862, #6363, #7876, #7695, #8754, #23029, #5969 ) ) ;
#15026=EDGE_CURVE ( 'NONE', #6791, #9879, #8905, .T. ) ;
#15031=FACE_OUTER_BOUND ( 'NONE', #877, .T. ) ;
#15042=CARTESIAN_POINT ( 'NONE',  ( 151.4000000000000057, -3695.699999999999818, 2296.591799999999694 ) ) ;
#15057=DIRECTION ( 'NONE',  ( 0.000000000000000000, 1.000000000000000000, 0.000000000000000000 ) ) ;
#15064=VECTOR ( 'NONE', #9897, 1000.000000000000000 ) ;
#15072=ORIENTED_EDGE ( 'NONE', *, *, #16803, .T. ) ;
#15076=FACE_BOUND ( 'NONE', #8903, .T. ) ;
#15077=CARTESIAN_POINT ( 'NONE',  ( 60.73942059830999796, -3544.061999999999898, 2279.618249568000010 ) ) ;
#15103=VECTOR ( 'NONE', #18492, 1000.000000000000000 ) ;
#15116=ORIENTED_EDGE ( 'NONE', *, *, #13282, .F. ) ;
#15120=ORIENTED_EDGE ( 'NONE', *, *, #7128, .F. ) ;
#15130=PLANE ( 'NONE',  #14508 ) ;
#15142=EDGE_LOOP ( 'NONE', ( #12039, #19474, #1614, #14524, #1533, #13460, #7192, #9305, #8828, #13785, #13335 ) ) ;
#15143=AXIS2_PLACEMENT_3D ( 'NONE', #3233, #17638, #19294 ) ;
#15145=CARTESIAN_POINT ( 'NONE',  ( 6.223000000000999066, -3599.497499999999945, 2295.829799999999977 ) ) ;
#15149=DIRECTION ( 'NONE',  ( -0.7071067811865693331, 0.000000000000000000, 0.7071067811865257013 ) ) ;
#15153=SHAPE_REPRESENTATION_RELATIONSHIP ( 'NONE' , 'NONE' ,  #1421, #7671 ) ;
#15157=CARTESIAN_POINT ( 'NONE',  ( 0.7620000000000000107, -3695.699999999999818, 2275.763800000000174 ) ) ;
#15163=CARTESIAN_POINT ( 'NONE',  ( 22.54063073453000143, -3544.061999999999898, 2275.763800000000174 ) ) ;
#15190=DIRECTION ( 'NONE',  ( 0.000000000000000000, -1.000000000000000000, 0.000000000000000000 ) ) ;
#15197=DIRECTION ( 'NONE',  ( 0.000000000000000000, 0.000000000000000000, -1.000000000000000000 ) ) ;
#15199=ORIENTED_EDGE ( 'NONE', *, *, #6061, .T. ) ;
#15224=ADVANCED_FACE ( 'NONE', ( #10162 ), #14323, .T. ) ;
#15229=EDGE_CURVE ( 'NONE', #19560, #7880, #8537, .T. ) ;
#15238=VERTEX_POINT ( 'NONE', #8643 ) ;
#15261=ORIENTED_EDGE ( 'NONE', *, *, #8263, .T. ) ;
#15308=ADVANCED_FACE ( 'NONE', ( #19311 ), #2904, .T. ) ;
#15322=CARTESIAN_POINT ( 'NONE',  ( 12.69999999999999929, -3599.497499999999945, 2295.829799999999977 ) ) ;
#15357=DIRECTION ( 'NONE',  ( 0.7249994335945011414, 0.000000000000000000, 0.6887494619146010688 ) ) ;
#15359=AXIS2_PLACEMENT_3D ( 'NONE', #13343, #17427, #19078 ) ;
#15367=CIRCLE ( 'NONE', #19859, 0.7619999999999554907 ) ;
#15380=DIRECTION ( 'NONE',  ( 0.7071067811865969777, 0.000000000000000000, 0.7071067811864980568 ) ) ;
#15385=ADVANCED_FACE ( 'NONE', ( #7357 ), #10980, .F. ) ;
#15386=DIRECTION ( 'NONE',  ( 0.000000000000000000, 1.000000000000000000, 0.000000000000000000 ) ) ;
#15389=CARTESIAN_POINT ( 'NONE',  ( 152.4000000000000057, -3694.938000000000102, 2275.763800000000174 ) ) ;
#15397=ORIENTED_EDGE ( 'NONE', *, *, #22996, .T. ) ;
#15401=CARTESIAN_POINT ( 'NONE',  ( 3.175000000094025054, -3694.938000000000102, 2275.001800000090952 ) ) ;
#15402=AXIS2_PLACEMENT_3D ( 'NONE', #1426, #12327, #19471 ) ;
#15437=CARTESIAN_POINT ( 'NONE',  ( 22.54063073453000143, -3544.061999999999898, 2275.763800000000174 ) ) ;
#15443=ORIENTED_EDGE ( 'NONE', *, *, #21710, .T. ) ;
#15455=SPHERICAL_SURFACE ( 'NONE', #18483, 0.7620000000000000107 ) ;
#15479=VECTOR ( 'NONE', #8933, 1000.000000000000000 ) ;
#15485=ORIENTED_EDGE ( 'NONE', *, *, #21138, .T. ) ;
#15491=DIRECTION ( 'NONE',  ( 1.000000000000000000, 0.000000000000000000, 0.000000000000000000 ) ) ;
#15513=ORIENTED_EDGE ( 'NONE', *, *, #3000, .T. ) ;
#15518=DIRECTION ( 'NONE',  ( 0.7071067811865969777, 0.000000000000000000, 0.7071067811864980568 ) ) ;
#15531=ORIENTED_EDGE ( 'NONE', *, *, #4938, .F. ) ;
#15546=PRODUCT ( 'Magnet Chuck Plate', 'Magnet Chuck Plate', '', ( #10689 ) ) ;
#15556=DIRECTION ( 'NONE',  ( 0.000000000000000000, 0.000000000000000000, 1.000000000000000000 ) ) ;
#15575=CIRCLE ( 'NONE', #6968, 1.523999999999858801 ) ;
#15579=LINE ( 'NONE', #13937, #12553 ) ;
#15587=ORIENTED_EDGE ( 'NONE', *, *, #3430, .T. ) ;
#15601=DIRECTION ( 'NONE',  ( 1.000000000000000000, 0.000000000000000000, 0.000000000000000000 ) ) ;
#15602=EDGE_CURVE ( 'NONE', #14578, #13412, #16880, .T. ) ;
#15604=CIRCLE ( 'NONE', #5137, 2.844800000000091700 ) ;
#15621=CARTESIAN_POINT ( 'NONE',  ( 2.859369265473000077, -3695.699999999999818, 2275.763800000000174 ) ) ;
#15624=DIRECTION ( 'NONE',  ( 0.000000000000000000, 0.000000000000000000, 1.000000000000000000 ) ) ;
#15644=ORIENTED_EDGE ( 'NONE', *, *, #19899, .T. ) ;
#15645=DIRECTION ( 'NONE',  ( 0.000000000000000000, 0.000000000000000000, 1.000000000000000000 ) ) ;
#15657=EDGE_CURVE ( 'NONE', #9083, #8878, #5305, .T. ) ;
#15660=ORIENTED_EDGE ( 'NONE', *, *, #9995, .T. ) ;
#15667=CYLINDRICAL_SURFACE ( 'NONE', #9201, 2.844800000000091700 ) ;
#15675=DIRECTION ( 'NONE',  ( 0.000000000000000000, 0.000000000000000000, 1.000000000000000000 ) ) ;
#15681=DIRECTION ( 'NONE',  ( 0.000000000000000000, 0.000000000000000000, -1.000000000000000000 ) ) ;
#15690=DIRECTION ( 'NONE',  ( 1.000000000000000000, 0.000000000000000000, 0.000000000000000000 ) ) ;
#15695=ORIENTED_EDGE ( 'NONE', *, *, #7361, .T. ) ;
#15696=DIRECTION ( 'NONE',  ( 0.000000000000000000, -1.000000000000000000, 0.000000000000000000 ) ) ;
#15735=( GEOMETRIC_REPRESENTATION_CONTEXT ( 3 ) GLOBAL_UNCERTAINTY_ASSIGNED_CONTEXT ( ( #5748 ) ) GLOBAL_UNIT_ASSIGNED_CONTEXT ( ( #9985, #8009, #6259 ) ) REPRESENTATION_CONTEXT ( 'NONE', 'WORKASPACE' ) );
#15743=PRODUCT_DEFINITION_SHAPE ( 'NONE', 'NONE',  #9636 ) ;
#15759=DIRECTION ( 'NONE',  ( 0.000000000000000000, -1.000000000000000000, 0.000000000000000000 ) ) ;
#15776=AXIS2_PLACEMENT_3D ( 'NONE', #20088, #1918, #2162 ) ;
#15796=DIRECTION ( 'NONE',  ( 0.000000000000000000, 0.000000000000000000, -1.000000000000000000 ) ) ;
#15804=CIRCLE ( 'NONE', #12443, 2.844799999999999773 ) ;
#15838=AXIS2_PLACEMENT_3D ( 'NONE', #5057, #10442, #10087 ) ;
#15865=AXIS2_PLACEMENT_3D ( 'NONE', #3957, #20137, #10992 ) ;
#15873=DIRECTION ( 'NONE',  ( 6.341789985291834412E-14, 0.000000000000000000, 1.000000000000000000 ) ) ;
#15877=CYLINDRICAL_SURFACE ( 'NONE', #6847, 2.844800000000091700 ) ;
#15891=ADVANCED_FACE ( 'NONE', ( #4265 ), #2509, .T. ) ;
#15899=CARTESIAN_POINT ( 'NONE',  ( 0.7620000000000000107, -3694.938000000000102, 2296.591799999999694 ) ) ;
#15905=DIRECTION ( 'NONE',  ( 0.000000000000000000, 0.000000000000000000, 1.000000000000000000 ) ) ;
#15908=DIRECTION ( 'NONE',  ( 1.000000000000000000, 0.000000000000000000, 0.000000000000000000 ) ) ;
#15916=CARTESIAN_POINT ( 'NONE',  ( 61.26424768829000556, -3544.061999999999898, 2279.065800000000309 ) ) ;
#15924=CARTESIAN_POINT ( 'NONE',  ( 0.7620000000000000107, -3543.299999999999727, 2295.829799999999977 ) ) ;
#15927=FACE_OUTER_BOUND ( 'NONE', #17449, .T. ) ;
#15935=CARTESIAN_POINT ( 'NONE',  ( 55.57575231171000496, -3694.938000000000102, 2275.763800000000174 ) ) ;
#15959=EDGE_CURVE ( 'NONE', #9431, #9191, #16450, .T. ) ;
#15962=CARTESIAN_POINT ( 'NONE',  ( 20.32000000000000028, -3544.061999999999898, 2289.213099999999940 ) ) ;
#15968=CARTESIAN_POINT ( 'NONE',  ( 15.54479999999999862, -3639.502500000000055, 2288.971800000000258 ) ) ;
#15973=EDGE_CURVE ( 'NONE', #4104, #15991, #520, .T. ) ;
#15976=ADVANCED_FACE ( 'NONE', ( #16567 ), #16679, .T. ) ;
#15986=EDGE_LOOP ( 'NONE', ( #20064, #19332, #14244, #2134 ) ) ;
#15991=VERTEX_POINT ( 'NONE', #6616 ) ;
#16007=DIRECTION ( 'NONE',  ( 1.000000000000000000, 0.000000000000000000, 0.000000000000000000 ) ) ;
#16061=CARTESIAN_POINT ( 'NONE',  ( 0.7620000000000000107, -3694.938000000000102, 2275.763800000000174 ) ) ;
#16081=AXIS2_PLACEMENT_3D ( 'NONE', #14016, #1584, #5228 ) ;
#16112=CARTESIAN_POINT ( 'NONE',  ( 20.32000000000000028, -3694.938000000000102, 2286.368300000000090 ) ) ;
#16116=DIRECTION ( 'NONE',  ( -1.000000000000000000, 0.000000000000000000, 0.000000000000000000 ) ) ;
#16120=ORIENTED_EDGE ( 'NONE', *, *, #13042, .T. ) ;
#16123=CARTESIAN_POINT ( 'NONE',  ( 20.32000000000000028, -3694.938000000000102, 2289.213099999999940 ) ) ;
#16140=EDGE_CURVE ( 'NONE', #11162, #2445, #13157, .T. ) ;
#16158=CARTESIAN_POINT ( 'NONE',  ( 64.76999999999999602, -3543.299999999999727, 2285.606299999999919 ) ) ;
#16160=ADVANCED_FACE ( 'NONE', ( #3308 ), #12452, .T. ) ;
#16164=LINE ( 'NONE', #16277, #3066 ) ;
#16165=ORIENTED_EDGE ( 'NONE', *, *, #9000, .F. ) ;
#16181=LINE ( 'NONE', #3638, #17766 ) ;
#16189=AXIS2_PLACEMENT_3D ( 'NONE', #11925, #6669, #22804 ) ;
#16190=CARTESIAN_POINT ( 'NONE',  ( 15.87500000000000000, -3694.938000000000102, 2282.113800000000083 ) ) ;
#16192=ORIENTED_EDGE ( 'NONE', *, *, #10815, .T. ) ;
#16223=DIRECTION ( 'NONE',  ( 0.000000000000000000, 0.000000000000000000, 1.000000000000000000 ) ) ;
#16237=FACE_OUTER_BOUND ( 'NONE', #3901, .T. ) ;
#16242=VERTEX_POINT ( 'NONE', #15968 ) ;
#16250=ORIENTED_EDGE ( 'NONE', *, *, #21985, .F. ) ;
#16264=FACE_BOUND ( 'NONE', #19844, .T. ) ;
#16266=AXIS2_PLACEMENT_3D ( 'NONE', #10762, #12985, #18360 ) ;
#16277=CARTESIAN_POINT ( 'NONE',  ( 0.7620000000000000107, -3695.699999999999818, 2295.829799999999977 ) ) ;
#16297=CYLINDRICAL_SURFACE ( 'NONE', #2010, 2.844800000000091700 ) ;
#16334=EDGE_LOOP ( 'NONE', ( #3403, #16572, #9060, #12798 ) ) ;
#16337=EDGE_LOOP ( 'NONE', ( #4986, #6980, #11760, #14026 ) ) ;
#16371=CARTESIAN_POINT ( 'NONE',  ( 64.76999999999999602, -3568.700000000000273, 2289.213099999999940 ) ) ;
#16381=PLANE ( 'NONE',  #21856 ) ;
#16390=DIRECTION ( 'NONE',  ( 1.000000000000000000, 0.000000000000000000, 0.000000000000000000 ) ) ;
#16394=EDGE_LOOP ( 'NONE', ( #16768, #9062 ) ) ;
#16396=EDGE_CURVE ( 'NONE', #2028, #16242, #15804, .T. ) ;
#16415=AXIS2_PLACEMENT_3D ( 'NONE', #10038, #21185, #10155 ) ;
#16429=EDGE_CURVE ( 'NONE', #18286, #1414, #1736, .T. ) ;
#16436=EDGE_CURVE ( 'NONE', #7405, #10930, #4896, .T. ) ;
#16446=EDGE_CURVE ( 'NONE', #8260, #9227, #11667, .T. ) ;
#16450=LINE ( 'NONE', #9534, #6063 ) ;
#16493=LINE ( 'NONE', #14750, #12198 ) ;
#16499=ORIENTED_EDGE ( 'NONE', *, *, #211, .F. ) ;
#16502=ORIENTED_EDGE ( 'NONE', *, *, #22802, .T. ) ;
#16514=EDGE_LOOP ( 'NONE', ( #16912, #21085, #17914 ) ) ;
#16558=CARTESIAN_POINT ( 'NONE',  ( 55.57575231171000496, -3694.938000000000102, 2275.001800000000003 ) ) ;
#16565=AXIS2_PLACEMENT_3D ( 'NONE', #2175, #1819, #16116 ) ;
#16567=FACE_OUTER_BOUND ( 'NONE', #5345, .T. ) ;
#16569=VECTOR ( 'NONE', #1428, 1000.000000000000000 ) ;
#16572=ORIENTED_EDGE ( 'NONE', *, *, #7072, .F. ) ;
#16575=DIRECTION ( 'NONE',  ( 0.000000000000000000, 0.000000000000000000, 1.000000000000000000 ) ) ;
#16611=VECTOR ( 'NONE', #8548, 1000.000000000000000 ) ;
#16615=CARTESIAN_POINT ( 'NONE',  ( 9.855199999999999960, -3639.502500000000055, 2288.971800000000258 ) ) ;
#16617=CARTESIAN_POINT ( 'NONE',  ( 151.4000000000000057, -3695.699999999999818, 2275.001800000000003 ) ) ;
#16618=VERTEX_POINT ( 'NONE', #21541 ) ;
#16626=AXIS2_PLACEMENT_3D ( 'NONE', #4399, #20339, #8029 ) ;
#16628=ORIENTED_EDGE ( 'NONE', *, *, #2824, .F. ) ;
#16655=EDGE_CURVE ( 'NONE', #22767, #2058, #19547, .T. ) ;
#16666=ORIENTED_EDGE ( 'NONE', *, *, #4938, .T. ) ;
#16672=LINE ( 'NONE', #17130, #12477 ) ;
#16675=CARTESIAN_POINT ( 'NONE',  ( 64.76999999999999602, -3568.700000000000273, 2289.213099999999940 ) ) ;
#16679=CYLINDRICAL_SURFACE ( 'NONE', #21024, 0.7619999999998753326 ) ;
#16682=ADVANCED_FACE ( 'NONE', ( #18587, #15076, #7814 ), #17046, .F. ) ;
#16685=AXIS2_PLACEMENT_3D ( 'NONE', #16765, #599, #13130 ) ;
#16697=ORIENTED_EDGE ( 'NONE', *, *, #2199, .F. ) ;
#16700=EDGE_CURVE ( 'NONE', #16884, #22365, #7925, .T. ) ;
#16701=FACE_OUTER_BOUND ( 'NONE', #17854, .T. ) ;
#16731=CIRCLE ( 'NONE', #2515, 0.7619999999999294005 ) ;
#16732=EDGE_LOOP ( 'NONE', ( #10786, #5808, #10210, #21694 ) ) ;
#16738=EDGE_CURVE ( 'NONE', #17590, #19948, #4956, .T. ) ;
#16741=UNCERTAINTY_MEASURE_WITH_UNIT (LENGTH_MEASURE( 1.000000000000000082E-05 ), #21126, 'distance_accuracy_value', 'NONE');
#16765=CARTESIAN_POINT ( 'NONE',  ( 12.69999999999999929, -3599.497499999999945, 2288.971800000000258 ) ) ;
#16768=ORIENTED_EDGE ( 'NONE', *, *, #15657, .T. ) ;
#16786=CARTESIAN_POINT ( 'NONE',  ( 0.7620000000000000107, -3694.938000000000102, 2295.829799999999977 ) ) ;
#16803=EDGE_CURVE ( 'NONE', #18833, #22793, #20563, .T. ) ;
#16828=DIRECTION ( 'NONE',  ( 0.000000000000000000, -1.000000000000000000, 0.000000000000000000 ) ) ;
#16861=CARTESIAN_POINT ( 'NONE',  ( 20.32000000000000028, -3543.299999999999727, 2285.606299999999919 ) ) ;
#16865=ORIENTED_EDGE ( 'NONE', *, *, #18597, .F. ) ;
#16875=CARTESIAN_POINT ( 'NONE',  ( 0.7620000000000000107, -3694.938000000000102, 2295.829799999999977 ) ) ;
#16880=CIRCLE ( 'NONE', #21396, 0.7619999999999294005 ) ;
#16884=VERTEX_POINT ( 'NONE', #14486 ) ;
#16897=DIRECTION ( 'NONE',  ( -1.224646799147353207E-16, 1.000000000000000000, 0.000000000000000000 ) ) ;
#16903=FACE_OUTER_BOUND ( 'NONE', #20027, .T. ) ;
#16912=ORIENTED_EDGE ( 'NONE', *, *, #9941, .T. ) ;
#16916=ORIENTED_EDGE ( 'NONE', *, *, #17738, .T. ) ;
#16918=CARTESIAN_POINT ( 'NONE',  ( 64.76999999999999602, -3670.300000000000182, 2289.213099999999940 ) ) ;
#16931=DIRECTION ( 'NONE',  ( -1.000000000000000000, 0.000000000000000000, 0.000000000000000000 ) ) ;
#16933=CARTESIAN_POINT ( 'NONE',  ( 16.19063073439513190, -3543.299999999999727, 2282.113800000000083 ) ) ;
#16936=CIRCLE ( 'NONE', #21826, 0.7619999999999294005 ) ;
#16946=LINE ( 'NONE', #17762, #21192 ) ;
#16954=EDGE_CURVE ( 'NONE', #20566, #18833, #21511, .T. ) ;
#16962=CLOSED_SHELL ( 'NONE', ( #16968, #10228, #11009, #4329, #255, #13757, #14186, #18686, #3539, #19041, #254, #8489, #9795, #13546, #11850, #13576, #16682, #3410, #18661, #17852, #23051, #7632, #15224, #11356, #18750, #2202, #1325, #11422, #2511, #8846, #15385, #11832, #21041, #20414, #19896, #355, #11949, #21621, #14882, #15976, #1261, #18586, #6374, #8948, #661, #21196, #116, #20707, #15308, #8218, #18324, #19167, #4994, #942, #13635, #17595, #9531, #851, #13672, #21833, #5165, #14170, #3716, #13391, #10552, #6750, #18446, #19091, #17225, #10726, #15891, #11363, #12930, #3120, #6213, #18615, #6884, #22549, #16160 ) ) ;
#16968=ADVANCED_FACE ( 'NONE', ( #7551 ), #460, .T. ) ;
#16975=ORIENTED_EDGE ( 'NONE', *, *, #6706, .F. ) ;
#16988=CIRCLE ( 'NONE', #18848, 0.7619999999999294005 ) ;
#17005=VECTOR ( 'NONE', #7539, 1000.000000000000000 ) ;
#17020=CARTESIAN_POINT ( 'NONE',  ( 9.209369265563442042, -3543.299999999999727, 2282.113800000095125 ) ) ;
#17027=ORIENTED_EDGE ( 'NONE', *, *, #7798, .T. ) ;
#17032=EDGE_LOOP ( 'NONE', ( #18032, #5092, #8222, #1626 ) ) ;
#17046=PLANE ( 'NONE',  #3077 ) ;
#17070=EDGE_CURVE ( 'NONE', #5647, #3812, #9096, .T. ) ;
#17091=CARTESIAN_POINT ( 'NONE',  ( 60.96000000000000085, -3543.299999999999727, 2279.827800000000025 ) ) ;
#17120=EDGE_LOOP ( 'NONE', ( #21853, #22334 ) ) ;
#17125=EDGE_LOOP ( 'NONE', ( #18276, #15443, #2732, #13236 ) ) ;
#17130=CARTESIAN_POINT ( 'NONE',  ( 0.000000000000000000, -3694.938000000000102, 2275.763800000000174 ) ) ;
#17146=ORIENTED_EDGE ( 'NONE', *, *, #3981, .F. ) ;
#17156=CARTESIAN_POINT ( 'NONE',  ( 12.69999999999999929, -3599.497499999999945, 2288.971800000000258 ) ) ;
#17160=DIRECTION ( 'NONE',  ( 0.000000000000000000, -1.000000000000000000, 0.000000000000000000 ) ) ;
#17173=VECTOR ( 'NONE', #15905, 1000.000000000000000 ) ;
#17207=ORIENTED_EDGE ( 'NONE', *, *, #16436, .T. ) ;
#17217=DIRECTION ( 'NONE',  ( 0.6887494619147179753, 0.000000000000000000, -0.7249994335943901191 ) ) ;
#17225=ADVANCED_FACE ( 'NONE', ( #12339 ), #1794, .T. ) ;
#17243=CARTESIAN_POINT ( 'NONE',  ( 0.000000000000000000, -3694.938000000000102, 2295.829799999999977 ) ) ;
#17263=DIRECTION ( 'NONE',  ( 0.000000000000000000, 0.000000000000000000, 1.000000000000000000 ) ) ;
#17268=LINE ( 'NONE', #17373, #250 ) ;
#17270=DIRECTION ( 'NONE',  ( -1.000000000000000000, 0.000000000000000000, 0.000000000000000000 ) ) ;
#17278=DIRECTION ( 'NONE',  ( 0.000000000000000000, 0.000000000000000000, -1.000000000000000000 ) ) ;
#17283=CARTESIAN_POINT ( 'NONE',  ( 12.69999999999999929, -3599.497499999999945, 2263.571799999999712 ) ) ;
#17321=ORIENTED_EDGE ( 'NONE', *, *, #4101, .F. ) ;
#17324=VECTOR ( 'NONE', #12425, 1000.000000000000000 ) ;
#17366=AXIS2_PLACEMENT_3D ( 'NONE', #14775, #13124, #18054 ) ;
#17373=CARTESIAN_POINT ( 'NONE',  ( 151.6380000000000052, -3695.699999999999818, 2280.589800000000196 ) ) ;
#17379=CIRCLE ( 'NONE', #194, 1.523999999999965160 ) ;
#17381=AXIS2_PLACEMENT_3D ( 'NONE', #8864, #16007, #7222 ) ;
#17384=ORIENTED_EDGE ( 'NONE', *, *, #1847, .F. ) ;
#17389=AXIS2_PLACEMENT_3D ( 'NONE', #6137, #22393, #6365 ) ;
#17395=CARTESIAN_POINT ( 'NONE',  ( 0.7620000000000000107, -3694.938000000000102, 2275.001800000000003 ) ) ;
#17403=VECTOR ( 'NONE', #13557, 1000.000000000000114 ) ;
#17427=DIRECTION ( 'NONE',  ( 0.000000000000000000, -1.000000000000000000, 0.000000000000000000 ) ) ;
#17430=AXIS2_PLACEMENT_3D ( 'NONE', #1940, #9092, #12137 ) ;
#17432=FACE_OUTER_BOUND ( 'NONE', #9701, .T. ) ;
#17441=CARTESIAN_POINT ( 'NONE',  ( 0.000000000000000000, -3544.061999999999898, 2295.829799999999977 ) ) ;
#17449=EDGE_LOOP ( 'NONE', ( #12254, #6413, #225, #22624 ) ) ;
#17453=SPHERICAL_SURFACE ( 'NONE', #4571, 0.7620000000000000107 ) ;
#17463=EDGE_LOOP ( 'NONE', ( #12814, #4349 ) ) ;
#17465=AXIS2_PLACEMENT_3D ( 'NONE', #12342, #7189, #3313 ) ;
#17471=EDGE_CURVE ( 'NONE', #16618, #1484, #19579, .T. ) ;
#17472=DIRECTION ( 'NONE',  ( 1.000000000000000000, 0.000000000000000000, 0.000000000000000000 ) ) ;
#17474=FACE_OUTER_BOUND ( 'NONE', #19985, .T. ) ;
#17484=CIRCLE ( 'NONE', #19744, 0.7619999999999294005 ) ;
#17493=ORIENTED_EDGE ( 'NONE', *, *, #12076, .F. ) ;
#17495=CIRCLE ( 'NONE', #20492, 5.714999999998998881 ) ;
#17504=LINE ( 'NONE', #8842, #11823 ) ;
#17506=CYLINDRICAL_SURFACE ( 'NONE', #10339, 0.7619999999999294005 ) ;
#17533=EDGE_CURVE ( 'NONE', #14578, #5209, #17575, .T. ) ;
#17534=CARTESIAN_POINT ( 'NONE',  ( 20.32000000000000028, -3670.300000000000182, 2292.057900000000245 ) ) ;
#17566=ORIENTED_EDGE ( 'NONE', *, *, #18717, .F. ) ;
#17575=LINE ( 'NONE', #3741, #17324 ) ;
#17590=VERTEX_POINT ( 'NONE', #7053 ) ;
#17595=ADVANCED_FACE ( 'NONE', ( #7609 ), #18089, .T. ) ;
#17629=ORIENTED_EDGE ( 'NONE', *, *, #10371, .F. ) ;
#17638=DIRECTION ( 'NONE',  ( 0.000000000000000000, 1.000000000000000000, 0.000000000000000000 ) ) ;
#17656=DIRECTION ( 'NONE',  ( -1.000000000000000000, -0.000000000000000000, -0.000000000000000000 ) ) ;
#17681=FACE_OUTER_BOUND ( 'NONE', #21287, .T. ) ;
#17687=EDGE_CURVE ( 'NONE', #11834, #11029, #9117, .T. ) ;
#17691=CARTESIAN_POINT ( 'NONE',  ( 9.525000000092171959, -3544.061999999999898, 2281.351800000095409 ) ) ;
#17714=CIRCLE ( 'NONE', #19976, 0.7619999999999294005 ) ;
#17727=EDGE_CURVE ( 'NONE', #11029, #22409, #13978, .T. ) ;
#17728=ORIENTED_EDGE ( 'NONE', *, *, #10647, .T. ) ;
#17738=EDGE_CURVE ( 'NONE', #8260, #4017, #16936, .T. ) ;
#17750=AXIS2_PLACEMENT_3D ( 'NONE', #3960, #20140, #11115 ) ;
#17762=CARTESIAN_POINT ( 'NONE',  ( 15.87500000000000000, -3544.061999999999898, 2281.351799999999912 ) ) ;
#17766=VECTOR ( 'NONE', #19706, 1000.000000000000000 ) ;
#17767=FACE_OUTER_BOUND ( 'NONE', #16337, .T. ) ;
#17778=CARTESIAN_POINT ( 'NONE',  ( 15.87500000000000000, -3544.061999999999898, 2281.351799999999912 ) ) ;
#17780=DIRECTION ( 'NONE',  ( 1.000000000000000000, 0.000000000000000000, 0.000000000000000000 ) ) ;
#17793=ORIENTED_EDGE ( 'NONE', *, *, #13807, .F. ) ;
#17827=DIRECTION ( 'NONE',  ( 0.000000000000000000, 0.000000000000000000, -1.000000000000000000 ) ) ;
#17830=CARTESIAN_POINT ( 'NONE',  ( 0.7620000000000000107, -3695.699999999999818, 2295.829799999999977 ) ) ;
#17834=DIRECTION ( 'NONE',  ( 0.000000000000000000, -1.000000000000000000, 0.000000000000000000 ) ) ;
#17835=LINE ( 'NONE', #1219, #15479 ) ;
#17852=ADVANCED_FACE ( 'NONE', ( #17432 ), #4665, .T. ) ;
#17854=EDGE_LOOP ( 'NONE', ( #16499, #2695, #16250, #9576 ) ) ;
#17867=DIRECTION ( 'NONE',  ( 1.000000000000000000, 0.000000000000000000, 0.000000000000000000 ) ) ;
#17905=VERTEX_POINT ( 'NONE', #9207 ) ;
#17906=LINE ( 'NONE', #14631, #11736 ) ;
#17909=DIRECTION ( 'NONE',  ( 0.000000000000000000, -1.000000000000000000, 0.000000000000000000 ) ) ;
#17914=ORIENTED_EDGE ( 'NONE', *, *, #17471, .T. ) ;
#17929=DIRECTION ( 'NONE',  ( 0.000000000000000000, 1.000000000000000000, 0.000000000000000000 ) ) ;
#17934=DIRECTION ( 'NONE',  ( 1.000000000000000000, 0.000000000000000000, 0.000000000000000000 ) ) ;
#17941=CARTESIAN_POINT ( 'NONE',  ( 152.4000000000000057, -3695.699999999999818, 2296.591799999999694 ) ) ;
#17943=DIRECTION ( 'NONE',  ( 0.000000000000000000, 0.000000000000000000, -1.000000000000000000 ) ) ;
#17950=DIRECTION ( 'NONE',  ( 0.000000000000000000, 1.000000000000000000, 0.000000000000000000 ) ) ;
#17957=DIRECTION ( 'NONE',  ( 0.000000000000000000, 0.000000000000000000, 1.000000000000000000 ) ) ;
#17987=DIRECTION ( 'NONE',  ( -1.000000000000000000, -0.000000000000000000, -0.000000000000000000 ) ) ;
#17991=DIRECTION ( 'NONE',  ( 0.000000000000000000, 0.000000000000000000, 1.000000000000000000 ) ) ;
#18013=CARTESIAN_POINT ( 'NONE',  ( 64.76999999999999602, -3568.700000000000273, 2286.368300000000090 ) ) ;
#18017=CARTESIAN_POINT ( 'NONE',  ( 18.41499999999999915, -3639.502500000000055, 2295.829799999999977 ) ) ;
#18022=EDGE_CURVE ( 'NONE', #18622, #4922, #17835, .T. ) ;
#18023=CARTESIAN_POINT ( 'NONE',  ( 64.76999999999999602, -3670.300000000000182, 2286.368300000000090 ) ) ;
#18032=ORIENTED_EDGE ( 'NONE', *, *, #19335, .F. ) ;
#18053=ORIENTED_EDGE ( 'NONE', *, *, #13811, .F. ) ;
#18054=DIRECTION ( 'NONE',  ( 0.000000000000000000, 0.000000000000000000, 1.000000000000000000 ) ) ;
#18072=ORIENTED_EDGE ( 'NONE', *, *, #8810, .F. ) ;
#18073=DIRECTION ( 'NONE',  ( 0.000000000000000000, 1.000000000000000000, 0.000000000000000000 ) ) ;
#18085=ORIENTED_EDGE ( 'NONE', *, *, #16429, .F. ) ;
#18087=FACE_OUTER_BOUND ( 'NONE', #20074, .T. ) ;
#18089=TOROIDAL_SURFACE ( 'NONE', #14353, 3.606799999999999784, 0.7620000000000000107 ) ;
#18118=DIRECTION ( 'NONE',  ( -1.000000000000000000, 0.000000000000000000, 0.000000000000000000 ) ) ;
#18127=CARTESIAN_POINT ( 'NONE',  ( 55.57575231171000496, -3695.699999999999818, 2275.763800000000174 ) ) ;
#18133=ORIENTED_EDGE ( 'NONE', *, *, #16140, .T. ) ;
#18153=VECTOR ( 'NONE', #6106, 1000.000000000000000 ) ;
#18168=FACE_OUTER_BOUND ( 'NONE', #16732, .T. ) ;
#18185=DIRECTION ( 'NONE',  ( 0.000000000000000000, 0.000000000000000000, 1.000000000000000000 ) ) ;
#18187=ORIENTED_EDGE ( 'NONE', *, *, #7962, .T. ) ;
#18192=AXIS2_PLACEMENT_3D ( 'NONE', #7132, #14280, #17780 ) ;
#18196=CIRCLE ( 'NONE', #5483, 0.7619999999999294005 ) ;
#18203=DIRECTION ( 'NONE',  ( -0.000000000000000000, 1.000000000000000000, 0.000000000000000000 ) ) ;
#18225=CARTESIAN_POINT ( 'NONE',  ( 15.87499999990501287, -3694.938000000000102, 2281.351800000094954 ) ) ;
#18226=DIRECTION ( 'NONE',  ( 0.000000000000000000, 1.000000000000000000, 0.000000000000000000 ) ) ;
#18232=CARTESIAN_POINT ( 'NONE',  ( 12.69999999999999929, -3639.502500000000055, 2281.351799999999912 ) ) ;
#18250=DIRECTION ( 'NONE',  ( 1.730170395987526852E-13, -1.000000000000000000, 0.000000000000000000 ) ) ;
#18261=DIRECTION ( 'NONE',  ( -0.000000000000000000, 0.000000000000000000, 1.000000000000000000 ) ) ;
#18262=EDGE_CURVE ( 'NONE', #6249, #4922, #12487, .T. ) ;
#18268=CIRCLE ( 'NONE', #8171, 0.7619999999999294005 ) ;
#18270=DIRECTION ( 'NONE',  ( 0.000000000000000000, 0.000000000000000000, 1.000000000000000000 ) ) ;
#18276=ORIENTED_EDGE ( 'NONE', *, *, #8557, .F. ) ;
#18282=EDGE_LOOP ( 'NONE', ( #11648, #5540, #10166, #6969 ) ) ;
#18283=AXIS2_PLACEMENT_3D ( 'NONE', #400, #5804, #2279 ) ;
#18284=DIRECTION ( 'NONE',  ( 0.000000000000000000, 0.000000000000000000, -1.000000000000000000 ) ) ;
#18286=VERTEX_POINT ( 'NONE', #5051 ) ;
#18288=CARTESIAN_POINT ( 'NONE',  ( 64.76999999999999602, -3568.700000000000273, 2289.213099999999940 ) ) ;
#18319=ORIENTED_EDGE ( 'NONE', *, *, #2424, .F. ) ;
#18320=FACE_OUTER_BOUND ( 'NONE', #14081, .T. ) ;
#18321=DIRECTION ( 'NONE',  ( -1.000000000000000000, -9.561467977825999598E-14, 0.000000000000000000 ) ) ;
#18323=CARTESIAN_POINT ( 'NONE',  ( 152.4000000000000057, -3544.061999999999898, 2275.763800000000174 ) ) ;
#18324=ADVANCED_FACE ( 'NONE', ( #18846 ), #15455, .T. ) ;
#18328=EDGE_LOOP ( 'NONE', ( #8147, #555, #7752, #20615 ) ) ;
#18344=CARTESIAN_POINT ( 'NONE',  ( 9.525000000266215849, -3543.615630734461320, 2281.351799999999912 ) ) ;
#18345=DIRECTION ( 'NONE',  ( -1.000000000000000000, -0.000000000000000000, -0.000000000000000000 ) ) ;
#18350=AXIS2_PLACEMENT_3D ( 'NONE', #4179, #9236, #440 ) ;
#18360=DIRECTION ( 'NONE',  ( 0.000000000000000000, 0.000000000000000000, -1.000000000000000000 ) ) ;
#18377=EDGE_CURVE ( 'NONE', #3900, #14108, #13226, .T. ) ;
#18389=DIRECTION ( 'NONE',  ( -1.000000000000000000, 0.000000000000000000, 0.000000000000000000 ) ) ;
#18392=AXIS2_PLACEMENT_3D ( 'NONE', #13783, #17278, #4863 ) ;
#18405=EDGE_CURVE ( 'NONE', #5100, #4633, #13819, .T. ) ;
#18436=DIRECTION ( 'NONE',  ( 0.000000000000000000, 1.000000000000000000, 0.000000000000000000 ) ) ;
#18446=ADVANCED_FACE ( 'NONE', ( #21204 ), #5257, .T. ) ;
#18449=CARTESIAN_POINT ( 'NONE',  ( 0.7620000000000000107, -3695.699999999999818, 2295.829799999999977 ) ) ;
#18461=VECTOR ( 'NONE', #12323, 1000.000000000000000 ) ;
#18466=ORIENTED_EDGE ( 'NONE', *, *, #15229, .T. ) ;
#18469=DIRECTION ( 'NONE',  ( -1.000000000000000000, 0.000000000000000000, 0.000000000000000000 ) ) ;
#18483=AXIS2_PLACEMENT_3D ( 'NONE', #18505, #6327, #13459 ) ;
#18492=DIRECTION ( 'NONE',  ( 0.000000000000000000, 0.000000000000000000, -1.000000000000000000 ) ) ;
#18494=DIRECTION ( 'NONE',  ( 0.000000000000000000, 1.000000000000000000, 0.000000000000000000 ) ) ;
#18504=CIRCLE ( 'NONE', #8408, 2.844800000000091700 ) ;
#18505=CARTESIAN_POINT ( 'NONE',  ( 0.7620000000000000107, -3694.938000000000102, 2295.829799999999977 ) ) ;
#18506=ORIENTED_EDGE ( 'NONE', *, *, #2776, .T. ) ;
#18510=VERTEX_POINT ( 'NONE', #15924 ) ;
#18518=EDGE_LOOP ( 'NONE', ( #7634, #7096, #19870, #10910 ) ) ;
#18524=ORIENTED_EDGE ( 'NONE', *, *, #17533, .T. ) ;
#18538=ORIENTED_EDGE ( 'NONE', *, *, #8221, .T. ) ;
#18544=ORIENTED_EDGE ( 'NONE', *, *, #22817, .F. ) ;
#18573=DIRECTION ( 'NONE',  ( 1.000000000000000000, 0.000000000000000000, 0.000000000000000000 ) ) ;
#18586=ADVANCED_FACE ( 'NONE', ( #9125 ), #7368, .F. ) ;
#18587=FACE_BOUND ( 'NONE', #6070, .T. ) ;
#18593=CARTESIAN_POINT ( 'NONE',  ( 12.69999999999999929, -3639.502500000000055, 2288.971800000000258 ) ) ;
#18595=CARTESIAN_POINT ( 'NONE',  ( 20.32000000000000028, -3544.061999999999898, 2289.213099999999940 ) ) ;
#18597=EDGE_CURVE ( 'NONE', #9312, #6119, #16988, .T. ) ;
#18615=ADVANCED_FACE ( 'NONE', ( #16264, #2207 ), #16381, .F. ) ;
#18619=DIRECTION ( 'NONE',  ( 0.000000000000000000, 0.000000000000000000, 1.000000000000000000 ) ) ;
#18622=VERTEX_POINT ( 'NONE', #18023 ) ;
#18633=ORIENTED_EDGE ( 'NONE', *, *, #17070, .T. ) ;
#18634=AXIS2_PLACEMENT_3D ( 'NONE', #15389, #18898, #6266 ) ;
#18639=ORIENTED_EDGE ( 'NONE', *, *, #5372, .F. ) ;
#18653=EDGE_CURVE ( 'NONE', #15991, #2058, #17906, .T. ) ;
#18661=ADVANCED_FACE ( 'NONE', ( #10875 ), #5614, .T. ) ;
#18686=ADVANCED_FACE ( 'NONE', ( #2761 ), #13632, .T. ) ;
#18699=DIRECTION ( 'NONE',  ( 0.000000000000000000, -1.000000000000000000, 0.000000000000000000 ) ) ;
#18717=EDGE_CURVE ( 'NONE', #8155, #10930, #5957, .T. ) ;
#18731=LINE ( 'NONE', #15003, #18153 ) ;
#18739=DIRECTION ( 'NONE',  ( 0.000000000000000000, 0.000000000000000000, -1.000000000000000000 ) ) ;
#18750=ADVANCED_FACE ( 'NONE', ( #6181, #6302 ), #13429, .F. ) ;
#18751=CARTESIAN_POINT ( 'NONE',  ( 20.32000000000000028, -3695.699999999999818, 2285.606299999999919 ) ) ;
#18756=AXIS2_PLACEMENT_3D ( 'NONE', #14580, #18203, #4027 ) ;
#18775=DIRECTION ( 'NONE',  ( -0.7249994335945011414, 0.000000000000000000, -0.6887494619146010688 ) ) ;
#18783=ORIENTED_EDGE ( 'NONE', *, *, #9138, .F. ) ;
#18792=ORIENTED_EDGE ( 'NONE', *, *, #5149, .F. ) ;
#18810=DIRECTION ( 'NONE',  ( 0.000000000000000000, -1.000000000000000000, 0.000000000000000000 ) ) ;
#18814=CYLINDRICAL_SURFACE ( 'NONE', #5481, 2.844799999999999773 ) ;
#18828=CARTESIAN_POINT ( 'NONE',  ( 9.209369265603214672, -3695.699999999999818, 2282.113800000000083 ) ) ;
#18833=VERTEX_POINT ( 'NONE', #19175 ) ;
#18836=EDGE_CURVE ( 'NONE', #9227, #8260, #1653, .T. ) ;
#18845=DIRECTION ( 'NONE',  ( 0.000000000000000000, 0.000000000000000000, -1.000000000000000000 ) ) ;
#18846=FACE_OUTER_BOUND ( 'NONE', #10610, .T. ) ;
#18848=AXIS2_PLACEMENT_3D ( 'NONE', #7586, #11112, #18250 ) ;
#18864=DIRECTION ( 'NONE',  ( -1.000000000000000000, 0.000000000000000000, 0.000000000000000000 ) ) ;
#18873=CARTESIAN_POINT ( 'NONE',  ( 61.26424768829000556, -3543.299999999999727, 2280.589800000000196 ) ) ;
#18888=DIRECTION ( 'NONE',  ( 0.000000000000000000, 1.000000000000000000, 0.000000000000000000 ) ) ;
#18892=DIRECTION ( 'NONE',  ( 0.000000000000000000, 1.000000000000000000, 0.000000000000000000 ) ) ;
#18897=ORIENTED_EDGE ( 'NONE', *, *, #22504, .T. ) ;
#18898=DIRECTION ( 'NONE',  ( 1.000000000000000000, 0.000000000000000000, 0.000000000000000000 ) ) ;
#18932=AXIS2_PLACEMENT_3D ( 'NONE', #4972, #15759, #15873 ) ;
#18933=ORIENTED_EDGE ( 'NONE', *, *, #7069, .F. ) ;
#18950=DIRECTION ( 'NONE',  ( 0.000000000000000000, 0.000000000000000000, -1.000000000000000000 ) ) ;
#18960=EDGE_LOOP ( 'NONE', ( #3297, #13485, #2377 ) ) ;
#18968=CARTESIAN_POINT ( 'NONE',  ( 61.26424768829000556, -3543.299999999999727, 2280.589800000000196 ) ) ;
#18970=CARTESIAN_POINT ( 'NONE',  ( 0.7620000000000000107, -3694.938000000000102, 2275.763800000000174 ) ) ;
#18972=CARTESIAN_POINT ( 'NONE',  ( 60.21459350832999746, -3543.299999999999727, 2280.170699136999701 ) ) ;
#18974=VECTOR ( 'NONE', #18270, 1000.000000000000000 ) ;
#18986=ORIENTED_EDGE ( 'NONE', *, *, #8557, .T. ) ;
#18999=CIRCLE ( 'NONE', #21986, 0.7619999999999294005 ) ;
#19004=CYLINDRICAL_SURFACE ( 'NONE', #6556, 0.7619999999999294005 ) ;
#19007=CIRCLE ( 'NONE', #8529, 3.606800000000021100 ) ;
#19026=EDGE_CURVE ( 'NONE', #1205, #17905, #415, .T. ) ;
#19041=ADVANCED_FACE ( 'NONE', ( #19764 ), #6940, .T. ) ;
#19043=CARTESIAN_POINT ( 'NONE',  ( 55.57575231171000496, -3543.299999999999727, 2275.763800000000174 ) ) ;
#19061=DIRECTION ( 'NONE',  ( 0.000000000000000000, 0.000000000000000000, -1.000000000000000000 ) ) ;
#19067=CYLINDRICAL_SURFACE ( 'NONE', #5341, 2.844799999999999773 ) ;
#19078=DIRECTION ( 'NONE',  ( 6.341789985291834412E-14, 0.000000000000000000, 1.000000000000000000 ) ) ;
#19083=DIRECTION ( 'NONE',  ( 0.000000000000000000, 0.000000000000000000, -1.000000000000000000 ) ) ;
#19085=VERTEX_POINT ( 'NONE', #14602 ) ;
#19091=ADVANCED_FACE ( 'NONE', ( #16237 ), #11191, .F. ) ;
#19134=FACE_OUTER_BOUND ( 'NONE', #8763, .T. ) ;
#19158=DIRECTION ( 'NONE',  ( -1.000000000000000000, 0.000000000000000000, 0.000000000000000000 ) ) ;
#19167=ADVANCED_FACE ( 'NONE', ( #22073 ), #19004, .T. ) ;
#19175=CARTESIAN_POINT ( 'NONE',  ( 22.54063073453000143, -3544.061999999999898, 2275.001800000000003 ) ) ;
#19190=LINE ( 'NONE', #17534, #4575 ) ;
#19210=EDGE_LOOP ( 'NONE', ( #701, #16865, #11887, #8669 ) ) ;
#19217=AXIS2_PLACEMENT_3D ( 'NONE', #2170, #18321, #295 ) ;
#19239=EDGE_LOOP ( 'NONE', ( #2521, #4449, #11333, #4536 ) ) ;
#19247=FACE_OUTER_BOUND ( 'NONE', #12260, .T. ) ;
#19267=CARTESIAN_POINT ( 'NONE',  ( 61.26424768829000556, -3695.699999999999818, 2279.065800000000309 ) ) ;
#19270=CARTESIAN_POINT ( 'NONE',  ( 8.986184632732999944, -3694.938000000000102, 2281.890615367000009 ) ) ;
#19293=CIRCLE ( 'NONE', #13295, 0.7619999999999294005 ) ;
#19294=DIRECTION ( 'NONE',  ( 0.000000000000000000, 0.000000000000000000, -1.000000000000000000 ) ) ;
#19298=CARTESIAN_POINT ( 'NONE',  ( 20.32000000000000028, -3670.300000000000182, 2289.213099999999940 ) ) ;
#19304=CYLINDRICAL_SURFACE ( 'NONE', #13313, 0.7619999999999294005 ) ;
#19305=DIRECTION ( 'NONE',  ( 0.000000000000000000, 0.000000000000000000, -1.000000000000000000 ) ) ;
#19307=DIRECTION ( 'NONE',  ( 1.000000000000000000, 0.000000000000000000, -1.224646799147353207E-16 ) ) ;
#19310=ORIENTED_EDGE ( 'NONE', *, *, #2924, .F. ) ;
#19311=FACE_OUTER_BOUND ( 'NONE', #12546, .T. ) ;
#19328=VERTEX_POINT ( 'NONE', #22616 ) ;
#19331=AXIS2_PLACEMENT_3D ( 'NONE', #12819, #23123, #5329 ) ;
#19332=ORIENTED_EDGE ( 'NONE', *, *, #9433, .T. ) ;
#19335=EDGE_CURVE ( 'NONE', #2445, #9572, #7276, .T. ) ;
#19351=CARTESIAN_POINT ( 'NONE',  ( 0.7620000000000000107, -3544.061999999999898, 2295.829799999999977 ) ) ;
#19355=DIRECTION ( 'NONE',  ( -0.000000000000000000, 1.000000000000000000, 0.000000000000000000 ) ) ;
#19359=DIRECTION ( 'NONE',  ( 0.000000000000000000, 0.000000000000000000, 1.000000000000000000 ) ) ;
#19366=CYLINDRICAL_SURFACE ( 'NONE', #626, 2.844799999999999773 ) ;
#19375=DIRECTION ( 'NONE',  ( 0.000000000000000000, -1.000000000000000000, 0.000000000000000000 ) ) ;
#19404=EDGE_CURVE ( 'NONE', #10059, #14578, #16181, .T. ) ;
#19405=VERTEX_POINT ( 'NONE', #7165 ) ;
#19471=DIRECTION ( 'NONE',  ( 0.000000000000000000, 0.000000000000000000, -1.000000000000000000 ) ) ;
#19474=ORIENTED_EDGE ( 'NONE', *, *, #1795, .F. ) ;
#19488=ORIENTED_EDGE ( 'NONE', *, *, #10647, .F. ) ;
#19491=ORIENTED_EDGE ( 'NONE', *, *, #11516, .T. ) ;
#19535=ORIENTED_EDGE ( 'NONE', *, *, #7069, .T. ) ;
#19547=CIRCLE ( 'NONE', #13551, 0.7619999999999294005 ) ;
#19560=VERTEX_POINT ( 'NONE', #2003 ) ;
#19574=CARTESIAN_POINT ( 'NONE',  ( 3.175000000265765010, -3543.615630734505430, 2275.001800000000003 ) ) ;
#19579=CIRCLE ( 'NONE', #3109, 0.7619999999999294005 ) ;
#19599=EDGE_CURVE ( 'NONE', #3230, #22409, #12778, .T. ) ;
#19639=ORIENTED_EDGE ( 'NONE', *, *, #7034, .F. ) ;
#19691=CIRCLE ( 'NONE', #9577, 2.844800000000091700 ) ;
#19697=CARTESIAN_POINT ( 'NONE',  ( 2.859369265602505816, -3543.299999999999727, 2275.763800000000629 ) ) ;
#19706=DIRECTION ( 'NONE',  ( 0.000000000000000000, -1.000000000000000000, 0.000000000000000000 ) ) ;
#19710=( BOUNDED_CURVE ( )  B_SPLINE_CURVE ( 3, ( #20003, #5941, #18344, #14844 ),
 .UNSPECIFIED., .F., .T. ) 
 B_SPLINE_CURVE_WITH_KNOTS ( ( 4, 4 ),
 ( 1.570796326606976656, 3.141592653589793116 ),
 .UNSPECIFIED. ) 
 CURVE ( )  GEOMETRIC_REPRESENTATION_ITEM ( )  RATIONAL_B_SPLINE_CURVE ( ( 1.000000000000000000, 0.8047378540800718127, 0.8047378540800718127, 1.000000000000000000 ) ) 
 REPRESENTATION_ITEM ( '' )  );
#19711=CARTESIAN_POINT ( 'NONE',  ( 152.4000000000000057, -3694.938000000000102, 2275.763800000000174 ) ) ;
#19719=DIRECTION ( 'NONE',  ( 0.000000000000000000, 1.000000000000000000, 0.000000000000000000 ) ) ;
#19726=CYLINDRICAL_SURFACE ( 'NONE', #9248, 5.715000000000001634 ) ;
#19744=AXIS2_PLACEMENT_3D ( 'NONE', #12862, #9462, #12982 ) ;
#19761=ORIENTED_EDGE ( 'NONE', *, *, #9271, .F. ) ;
#19764=FACE_OUTER_BOUND ( 'NONE', #13884, .T. ) ;
#19775=CIRCLE ( 'NONE', #1048, 3.606800000000021100 ) ;
#19782=CARTESIAN_POINT ( 'NONE',  ( 20.32000000000000028, -3543.299999999999727, 2289.213099999999940 ) ) ;
#19806=CARTESIAN_POINT ( 'NONE',  ( 56.10057940168000812, -3544.061999999999898, 2275.211350432000472 ) ) ;
#19821=CIRCLE ( 'NONE', #22789, 2.844799999999999773 ) ;
#19828=FACE_BOUND ( 'NONE', #3946, .T. ) ;
#19844=EDGE_LOOP ( 'NONE', ( #15397, #15485 ) ) ;
#19859=AXIS2_PLACEMENT_3D ( 'NONE', #21699, #9284, #7408 ) ;
#19870=ORIENTED_EDGE ( 'NONE', *, *, #7994, .F. ) ;
#19896=ADVANCED_FACE ( 'NONE', ( #15927 ), #9554, .T. ) ;
#19899=EDGE_CURVE ( 'NONE', #10930, #6730, #15579, .T. ) ;
#19909=LINE ( 'NONE', #13439, #17403 ) ;
#19940=CYLINDRICAL_SURFACE ( 'NONE', #14802, 0.7619999999999294005 ) ;
#19943=VECTOR ( 'NONE', #4056, 1000.000000000000000 ) ;
#19945=PLANE ( 'NONE',  #22456 ) ;
#19948=VERTEX_POINT ( 'NONE', #21084 ) ;
#19951=ORIENTED_EDGE ( 'NONE', *, *, #16700, .T. ) ;
#19952=AXIS2_PLACEMENT_3D ( 'NONE', #9891, #17160, #4289 ) ;
#19958=ORIENTED_EDGE ( 'NONE', *, *, #22461, .F. ) ;
#19967=CARTESIAN_POINT ( 'NONE',  ( 151.4000000000000057, -3694.938000000000102, 2296.591799999999694 ) ) ;
#19976=AXIS2_PLACEMENT_3D ( 'NONE', #8987, #18864, #2809 ) ;
#19985=EDGE_LOOP ( 'NONE', ( #8204, #10465, #2442, #9411 ) ) ;
#19998=ORIENTED_EDGE ( 'NONE', *, *, #13807, .T. ) ;
#20003=CARTESIAN_POINT ( 'NONE',  ( 9.209369265563442042, -3543.299999999999727, 2282.113800000095125 ) ) ;
#20010=EDGE_CURVE ( 'NONE', #2058, #19085, #16493, .T. ) ;
#20013=DIRECTION ( 'NONE',  ( 0.000000000000000000, 0.000000000000000000, -1.000000000000000000 ) ) ;
#20027=EDGE_LOOP ( 'NONE', ( #5993, #4708, #13692, #4316 ) ) ;
#20064=ORIENTED_EDGE ( 'NONE', *, *, #10815, .F. ) ;
#20065=DIRECTION ( 'NONE',  ( 0.000000000000000000, -1.000000000000000000, 0.000000000000000000 ) ) ;
#20069=EDGE_LOOP ( 'NONE', ( #5681, #9772, #21271, #13657 ) ) ;
#20074=EDGE_LOOP ( 'NONE', ( #2522, #11989 ) ) ;
#20083=AXIS2_PLACEMENT_3D ( 'NONE', #3275, #1513, #4525 ) ;
#20088=CARTESIAN_POINT ( 'NONE',  ( 12.69999999999999929, -3639.502500000000055, 2288.971800000000258 ) ) ;
#20095=CARTESIAN_POINT ( 'NONE',  ( 151.6380000000000052, -3694.938000000000102, 2296.591799999999694 ) ) ;
#20123=CARTESIAN_POINT ( 'NONE',  ( 0.7620000000000000107, -3543.299999999999727, 2295.829799999999977 ) ) ;
#20127=AXIS2_PLACEMENT_3D ( 'NONE', #8675, #15357, #17217 ) ;
#20137=DIRECTION ( 'NONE',  ( 0.000000000000000000, 1.000000000000000000, 0.000000000000000000 ) ) ;
#20140=DIRECTION ( 'NONE',  ( 0.000000000000000000, 0.000000000000000000, 1.000000000000000000 ) ) ;
#20143=DIRECTION ( 'NONE',  ( 0.000000000000000000, 1.000000000000000000, 0.000000000000000000 ) ) ;
#20172=ORIENTED_EDGE ( 'NONE', *, *, #7106, .F. ) ;
#20193=EDGE_CURVE ( 'NONE', #19328, #9572, #6220, .T. ) ;
#20203=CARTESIAN_POINT ( 'NONE',  ( 55.57575231171000496, -3695.699999999999818, 2275.763800000000174 ) ) ;
#20211=PLANE ( 'NONE',  #665 ) ;
#20223=CARTESIAN_POINT ( 'NONE',  ( 151.4000000000000057, -3543.299999999999727, 2280.589800000000196 ) ) ;
#20231=AXIS2_PLACEMENT_3D ( 'NONE', #14166, #8768, #12398 ) ;
#20236=EDGE_CURVE ( 'NONE', #7405, #9937, #16946, .T. ) ;
#20248=DIRECTION ( 'NONE',  ( 0.000000000000000000, -1.000000000000000000, 0.000000000000000000 ) ) ;
#20250=( BOUNDED_CURVE ( )  B_SPLINE_CURVE ( 3, ( #19697, #21678, #19574, #14195 ),
 .UNSPECIFIED., .F., .T. ) 
 B_SPLINE_CURVE_WITH_KNOTS ( ( 4, 4 ),
 ( 1.570796326731764836, 3.141592653589793116 ),
 .UNSPECIFIED. ) 
 CURVE ( )  GEOMETRIC_REPRESENTATION_ITEM ( )  RATIONAL_B_SPLINE_CURVE ( ( 1.000000000000000000, 0.8047378541094847293, 0.8047378541094847293, 1.000000000000000000 ) ) 
 REPRESENTATION_ITEM ( '' )  );
#20293=EDGE_CURVE ( 'NONE', #13309, #18286, #4877, .T. ) ;
#20299=EDGE_CURVE ( 'NONE', #6734, #1484, #3238, .T. ) ;
#20308=ORIENTED_EDGE ( 'NONE', *, *, #4675, .F. ) ;
#20315=CIRCLE ( 'NONE', #22170, 3.606800000000021100 ) ;
#20329=EDGE_LOOP ( 'NONE', ( #16975, #19761, #12251, #13383 ) ) ;
#20339=DIRECTION ( 'NONE',  ( -0.7071067811864976127, 0.000000000000000000, 0.7071067811865975328 ) ) ;
#20343=DIRECTION ( 'NONE',  ( 0.000000000000000000, 0.000000000000000000, -1.000000000000000000 ) ) ;
#20345=CARTESIAN_POINT ( 'NONE',  ( 64.76999999999999602, -3543.299999999999727, 2289.213099999999940 ) ) ;
#20350=DIRECTION ( 'NONE',  ( 0.000000000000000000, 0.000000000000000000, -1.000000000000000000 ) ) ;
#20358=DIRECTION ( 'NONE',  ( 0.000000000000000000, 0.000000000000000000, 1.000000000000000000 ) ) ;
#20360=CARTESIAN_POINT ( 'NONE',  ( 6.985000000000000320, -3639.502500000000055, 2288.971800000000258 ) ) ;
#20368=CARTESIAN_POINT ( 'NONE',  ( 16.19063073439513190, -3543.299999999999727, 2282.113800000000083 ) ) ;
#20375=TOROIDAL_SURFACE ( 'NONE', #180, 3.606799999999999784, 0.7620000000000000107 ) ;
#20377=DIRECTION ( 'NONE',  ( -0.7249994335945011414, 0.000000000000000000, -0.6887494619146010688 ) ) ;
#20394=CARTESIAN_POINT ( 'NONE',  ( 0.7620000000000000107, -3543.299999999999727, 2275.763800000000174 ) ) ;
#20403=CARTESIAN_POINT ( 'NONE',  ( 151.4000000000000057, -3695.699999999999818, 2280.589800000000196 ) ) ;
#20414=ADVANCED_FACE ( 'NONE', ( #5475 ), #5706, .F. ) ;
#20422=DIRECTION ( 'NONE',  ( 0.000000000000000000, -1.000000000000000000, 0.000000000000000000 ) ) ;
#20426=DIRECTION ( 'NONE',  ( -1.122008997397786234E-13, 0.000000000000000000, -1.000000000000000000 ) ) ;
#20442=AXIS2_PLACEMENT_3D ( 'NONE', #10830, #171, #21620 ) ;
#20444=EDGE_LOOP ( 'NONE', ( #15120, #14383, #4248, #3387 ) ) ;
#20453=CARTESIAN_POINT ( 'NONE',  ( 22.54063073453000143, -3694.938000000000102, 2275.001800000000003 ) ) ;
#20469=DIRECTION ( 'NONE',  ( 1.000000000000000000, 0.000000000000000000, 6.993530863773999741E-14 ) ) ;
#20476=CARTESIAN_POINT ( 'NONE',  ( 22.00181536726000076, -3694.938000000000102, 2275.224984633000076 ) ) ;
#20492=AXIS2_PLACEMENT_3D ( 'NONE', #20647, #20013, #8133 ) ;
#20495=CYLINDRICAL_SURFACE ( 'NONE', #5849, 2.844799999999999773 ) ;
#20526=ORIENTED_EDGE ( 'NONE', *, *, #22817, .T. ) ;
#20547=CARTESIAN_POINT ( 'NONE',  ( 55.57575231171000496, -3694.938000000000102, 2275.763800000000174 ) ) ;
#20549=PLANE ( 'NONE',  #16626 ) ;
#20563=LINE ( 'NONE', #9785, #13181 ) ;
#20566=VERTEX_POINT ( 'NONE', #1444 ) ;
#20570=CARTESIAN_POINT ( 'NONE',  ( 9.524999999998000177, -3694.938000000000102, 2281.351799999999912 ) ) ;
#20574=CARTESIAN_POINT ( 'NONE',  ( 2.859369265564648099, -3695.699999999999818, 2275.763800000091578 ) ) ;
#20575=CARTESIAN_POINT ( 'NONE',  ( 152.4000000000000057, -3695.699999999999818, 2275.001800000000003 ) ) ;
#20587=EDGE_CURVE ( 'NONE', #22767, #13412, #17379, .T. ) ;
#20604=CARTESIAN_POINT ( 'NONE',  ( 15.87499999990501287, -3694.938000000000102, 2281.351800000094954 ) ) ;
#20615=ORIENTED_EDGE ( 'NONE', *, *, #7834, .F. ) ;
#20635=ORIENTED_EDGE ( 'NONE', *, *, #16655, .T. ) ;
#20647=CARTESIAN_POINT ( 'NONE',  ( 12.69999999999999929, -3599.497499999999945, 2295.829799999999977 ) ) ;
#20650=DIRECTION ( 'NONE',  ( 0.000000000000000000, -1.000000000000000000, 0.000000000000000000 ) ) ;
#20651=CIRCLE ( 'NONE', #864, 0.7619999999999279572 ) ;
#20653=AXIS2_PLACEMENT_3D ( 'NONE', #10402, #14165, #15681 ) ;
#20656=VECTOR ( 'NONE', #15556, 1000.000000000000000 ) ;
#20662=VERTEX_POINT ( 'NONE', #14114 ) ;
#20686=DIRECTION ( 'NONE',  ( 1.000000000000000000, 0.000000000000000000, 3.680805717774999826E-13 ) ) ;
#20707=ADVANCED_FACE ( 'NONE', ( #22531 ), #6502, .T. ) ;
#20717=CARTESIAN_POINT ( 'NONE',  ( 20.32000000000000028, -3694.938000000000102, 2285.606299999999919 ) ) ;
#20734=EDGE_CURVE ( 'NONE', #4633, #7148, #10286, .T. ) ;
#20766=LINE ( 'NONE', #17243, #21448 ) ;
#20779=VERTEX_POINT ( 'NONE', #12812 ) ;
#20783=DIRECTION ( 'NONE',  ( -0.6887494619132868978, 0.000000000000000000, 0.7249994335957496983 ) ) ;
#20788=DIRECTION ( 'NONE',  ( -1.000000000000000000, 1.351868168142999859E-13, 0.000000000000000000 ) ) ;
#20799=VERTEX_POINT ( 'NONE', #19967 ) ;
#20804=VECTOR ( 'NONE', #12102, 1000.000000000000000 ) ;
#20808=LINE ( 'NONE', #15077, #6353 ) ;
#20819=CIRCLE ( 'NONE', #17430, 0.7619999999999294005 ) ;
#20822=AXIS2_PLACEMENT_3D ( 'NONE', #18595, #16828, #4417 ) ;
#20826=LINE ( 'NONE', #20476, #3569 ) ;
#20830=LINE ( 'NONE', #8410, #20656 ) ;
#20841=CYLINDRICAL_SURFACE ( 'NONE', #5474, 5.714999999998998881 ) ;
#20864=CARTESIAN_POINT ( 'NONE',  ( 55.57575231171000496, -3544.061999999999898, 2275.763800000000174 ) ) ;
#20880=CIRCLE ( 'NONE', #18283, 0.7619999999999987894 ) ;
#20882=CARTESIAN_POINT ( 'NONE',  ( 9.524999999997000089, -3544.061999999999898, 2281.351799999999912 ) ) ;
#20891=DIRECTION ( 'NONE',  ( 0.000000000000000000, 1.000000000000000000, 0.000000000000000000 ) ) ;
#20906=ORIENTED_EDGE ( 'NONE', *, *, #17687, .F. ) ;
#20934=AXIS2_PLACEMENT_3D ( 'NONE', #9223, #5600, #18118 ) ;
#20945=CARTESIAN_POINT ( 'NONE',  ( 64.76999999999999602, -3544.061999999999898, 2292.819899999999961 ) ) ;
#20973=EDGE_CURVE ( 'NONE', #7880, #9083, #19293, .T. ) ;
#21006=LINE ( 'NONE', #15621, #1134 ) ;
#21021=SPHERICAL_SURFACE ( 'NONE', #17465, 0.7620000000000000107 ) ;
#21024=AXIS2_PLACEMENT_3D ( 'NONE', #7658, #18775, #8132 ) ;
#21035=DIRECTION ( 'NONE',  ( 0.000000000000000000, 0.000000000000000000, -1.000000000000000000 ) ) ;
#21041=ADVANCED_FACE ( 'NONE', ( #1300 ), #22503, .T. ) ;
#21054=FACE_OUTER_BOUND ( 'NONE', #7375, .T. ) ;
#21064=CARTESIAN_POINT ( 'NONE',  ( 0.7620000000000000107, -3695.699999999999818, 2275.763800000000174 ) ) ;
#21065=DIRECTION ( 'NONE',  ( 0.000000000000000000, 0.000000000000000000, -1.000000000000000000 ) ) ;
#21080=DIRECTION ( 'NONE',  ( 1.000000000000000000, 0.000000000000000000, 0.000000000000000000 ) ) ;
#21084=CARTESIAN_POINT ( 'NONE',  ( 9.855199999999999960, -3639.502500000000055, 2281.351799999999912 ) ) ;
#21085=ORIENTED_EDGE ( 'NONE', *, *, #22900, .T. ) ;
#21086=CARTESIAN_POINT ( 'NONE',  ( 64.76999999999999602, -3544.061999999999898, 2286.368300000000090 ) ) ;
#21089=AXIS2_PLACEMENT_3D ( 'NONE', #4097, #4328, #18389 ) ;
#21095=FACE_OUTER_BOUND ( 'NONE', #5012, .T. ) ;
#21106=EDGE_CURVE ( 'NONE', #22211, #19405, #21237, .T. ) ;
#21110=DIRECTION ( 'NONE',  ( 0.000000000000000000, 0.000000000000000000, -1.000000000000000000 ) ) ;
#21119=FACE_OUTER_BOUND ( 'NONE', #9113, .T. ) ;
#21120=CARTESIAN_POINT ( 'NONE',  ( 12.69999999999999929, -3639.502500000000055, 2295.829799999999977 ) ) ;
#21121=AXIS2_PLACEMENT_3D ( 'NONE', #8657, #1743, #21080 ) ;
#21123=DIRECTION ( 'NONE',  ( 0.000000000000000000, 0.000000000000000000, 1.000000000000000000 ) ) ;
#21126=( LENGTH_UNIT ( ) NAMED_UNIT ( * ) SI_UNIT ( .MILLI., .METRE. ) );
#21138=EDGE_CURVE ( 'NONE', #20779, #17905, #11783, .T. ) ;
#21152=DIRECTION ( 'NONE',  ( -1.000000000000000000, 0.000000000000000000, 0.000000000000000000 ) ) ;
#21156=DIRECTION ( 'NONE',  ( -0.7071067811865975328, 0.000000000000000000, 0.7071067811864976127 ) ) ;
#21173=CARTESIAN_POINT ( 'NONE',  ( 12.69999999999999929, -3639.502500000000055, 2296.591799999999694 ) ) ;
#21185=DIRECTION ( 'NONE',  ( 1.000000000000000000, 0.000000000000000000, -1.224646799147353207E-16 ) ) ;
#21190=AXIS2_PLACEMENT_3D ( 'NONE', #4400, #753, #22421 ) ;
#21192=VECTOR ( 'NONE', #12379, 1000.000000000000000 ) ;
#21196=ADVANCED_FACE ( 'NONE', ( #5412 ), #14320, .T. ) ;
#21197=DIRECTION ( 'NONE',  ( -1.000000000000000000, 0.000000000000000000, 0.000000000000000000 ) ) ;
#21204=FACE_OUTER_BOUND ( 'NONE', #16334, .T. ) ;
#21219=DIRECTION ( 'NONE',  ( 0.6887494619147658259, 0.000000000000000000, -0.7249994335943447110 ) ) ;
#21232=AXIS2_PLACEMENT_3D ( 'NONE', #1589, #10383, #21404 ) ;
#21237=LINE ( 'NONE', #4939, #3192 ) ;
#21261=CIRCLE ( 'NONE', #1411, 0.7619999999999294005 ) ;
#21271=ORIENTED_EDGE ( 'NONE', *, *, #7543, .F. ) ;
#21287=EDGE_LOOP ( 'NONE', ( #2598, #15199, #21914 ) ) ;
#21302=ORIENTED_EDGE ( 'NONE', *, *, #17471, .F. ) ;
#21314=CIRCLE ( 'NONE', #1081, 0.7620000000000000107 ) ;
#21326=CARTESIAN_POINT ( 'NONE',  ( 64.76999999999999602, -3568.700000000000273, 2292.057900000000245 ) ) ;
#21352=CARTESIAN_POINT ( 'NONE',  ( 20.32000000000000028, -3670.300000000000182, 2289.213099999999940 ) ) ;
#21363=CARTESIAN_POINT ( 'NONE',  ( 20.32000000000000028, -3568.700000000000273, 2289.213099999999940 ) ) ;
#21394=CARTESIAN_POINT ( 'NONE',  ( 18.41499999999999915, -3639.502500000000055, 2288.971800000000258 ) ) ;
#21396=AXIS2_PLACEMENT_3D ( 'NONE', #11319, #18469, #14960 ) ;
#21404=DIRECTION ( 'NONE',  ( 0.000000000000000000, 0.000000000000000000, 1.000000000000000000 ) ) ;
#21407=DIRECTION ( 'NONE',  ( -1.000000000000000000, 0.000000000000000000, -3.680805717774999826E-13 ) ) ;
#21430=VECTOR ( 'NONE', #6551, 1000.000000000000000 ) ;
#21431=DIRECTION ( 'NONE',  ( 0.000000000000000000, 0.000000000000000000, 1.000000000000000000 ) ) ;
#21435=ORIENTED_EDGE ( 'NONE', *, *, #3000, .F. ) ;
#21442=EDGE_LOOP ( 'NONE', ( #11408, #5619, #2264, #14004 ) ) ;
#21446=CARTESIAN_POINT ( 'NONE',  ( 9.525000000260952504, -3695.384369265494115, 2281.351799999999912 ) ) ;
#21448=VECTOR ( 'NONE', #11312, 1000.000000000000000 ) ;
#21468=FACE_OUTER_BOUND ( 'NONE', #1933, .T. ) ;
#21471=DIRECTION ( 'NONE',  ( 0.000000000000000000, 0.000000000000000000, -1.000000000000000000 ) ) ;
#21488=CARTESIAN_POINT ( 'NONE',  ( 151.4000000000000057, -3695.699999999999818, 2295.829799999999977 ) ) ;
#21511=LINE ( 'NONE', #1702, #22892 ) ;
#21541=CARTESIAN_POINT ( 'NONE',  ( 0.7620000000000000107, -3543.299999999999727, 2275.763800000000174 ) ) ;
#21548=DIRECTION ( 'NONE',  ( 0.7249994335945980639, 0.000000000000000000, 0.6887494619144990393 ) ) ;
#21590=CARTESIAN_POINT ( 'NONE',  ( 20.32000000000000028, -3543.299999999999727, 2289.213099999999940 ) ) ;
#21620=DIRECTION ( 'NONE',  ( -0.6887494619136477203, 0.000000000000000000, 0.7249994335954068614 ) ) ;
#21621=ADVANCED_FACE ( 'NONE', ( #17767 ), #19304, .T. ) ;
#21628=VERTEX_POINT ( 'NONE', #20223 ) ;
#21635=DIRECTION ( 'NONE',  ( 0.000000000000000000, 1.000000000000000000, 0.000000000000000000 ) ) ;
#21647=ORIENTED_EDGE ( 'NONE', *, *, #9302, .T. ) ;
#21678=CARTESIAN_POINT ( 'NONE',  ( 3.044261469311703827, -3543.299999999971988, 2275.317430734553909 ) ) ;
#21694=ORIENTED_EDGE ( 'NONE', *, *, #18022, .F. ) ;
#21695=CARTESIAN_POINT ( 'NONE',  ( 151.4000000000000057, -3544.061999999999898, 2279.827800000000025 ) ) ;
#21699=CARTESIAN_POINT ( 'NONE',  ( 60.21459350834000190, -3544.061999999999898, 2280.170699136999701 ) ) ;
#21710=EDGE_CURVE ( 'NONE', #9431, #9937, #19710, .T. ) ;
#21749=ORIENTED_EDGE ( 'NONE', *, *, #762, .T. ) ;
#21759=ORIENTED_EDGE ( 'NONE', *, *, #4547, .T. ) ;
#21789=AXIS2_PLACEMENT_3D ( 'NONE', #11652, #9566, #16931 ) ;
#21802=ORIENTED_EDGE ( 'NONE', *, *, #19026, .F. ) ;
#21804=DIRECTION ( 'NONE',  ( 0.000000000000000000, -1.000000000000000000, 0.000000000000000000 ) ) ;
#21809=CIRCLE ( 'NONE', #13578, 0.7619999999999294005 ) ;
#21812=AXIS2_PLACEMENT_3D ( 'NONE', #8472, #21123, #3181 ) ;
#21826=AXIS2_PLACEMENT_3D ( 'NONE', #20717, #10053, #19083 ) ;
#21833=ADVANCED_FACE ( 'NONE', ( #14952 ), #13645, .T. ) ;
#21846=CYLINDRICAL_SURFACE ( 'NONE', #3277, 0.7619999999999294005 ) ;
#21849=DIRECTION ( 'NONE',  ( 0.000000000000000000, 0.000000000000000000, -1.000000000000000000 ) ) ;
#21853=ORIENTED_EDGE ( 'NONE', *, *, #13811, .T. ) ;
#21854=DIRECTION ( 'NONE',  ( 0.000000000000000000, -1.000000000000000000, 0.000000000000000000 ) ) ;
#21856=AXIS2_PLACEMENT_3D ( 'NONE', #7475, #14518, #14746 ) ;
#21858=DIRECTION ( 'NONE',  ( 0.000000000000000000, 0.000000000000000000, 1.000000000000000000 ) ) ;
#21871=EDGE_LOOP ( 'NONE', ( #17384, #17146, #6270, #3788, #18783, #1327, #3970, #18986, #16628, #11034, #18544 ) ) ;
#21896=ORIENTED_EDGE ( 'NONE', *, *, #21138, .F. ) ;
#21904=VECTOR ( 'NONE', #15696, 1000.000000000000000 ) ;
#21914=ORIENTED_EDGE ( 'NONE', *, *, #11576, .T. ) ;
#21931=CARTESIAN_POINT ( 'NONE',  ( 12.69999999999999929, -3639.502500000000055, 2288.971800000000258 ) ) ;
#21970=EDGE_CURVE ( 'NONE', #833, #5265, #22673, .T. ) ;
#21976=EDGE_CURVE ( 'NONE', #9879, #13412, #17268, .T. ) ;
#21985=EDGE_CURVE ( 'NONE', #4616, #8155, #17504, .T. ) ;
#21986=AXIS2_PLACEMENT_3D ( 'NONE', #441, #14966, #3834 ) ;
#21995=PLANE ( 'NONE',  #11063 ) ;
#22016=CARTESIAN_POINT ( 'NONE',  ( 22.00181536726000076, -3544.061999999999898, 2275.224984633000076 ) ) ;
#22042=AXIS2_PLACEMENT_3D ( 'NONE', #5344, #8512, #1703 ) ;
#22056=DIRECTION ( 'NONE',  ( -1.000000000000000000, 0.000000000000000000, 0.000000000000000000 ) ) ;
#22060=AXIS2_PLACEMENT_3D ( 'NONE', #14357, #12598, #17867 ) ;
#22071=CIRCLE ( 'NONE', #14247, 0.7619999999999294005 ) ;
#22073=FACE_OUTER_BOUND ( 'NONE', #22410, .T. ) ;
#22081=( BOUNDED_CURVE ( )  B_SPLINE_CURVE ( 3, ( #18225, #14495, #14720, #4048 ),
 .UNSPECIFIED., .F., .T. ) 
 B_SPLINE_CURVE_WITH_KNOTS ( ( 4, 4 ),
 ( 3.141592653589793116, 4.712388980572752573 ),
 .UNSPECIFIED. ) 
 CURVE ( )  GEOMETRIC_REPRESENTATION_ITEM ( )  RATIONAL_B_SPLINE_CURVE ( ( 1.000000000000000000, 0.8047378540800381730, 0.8047378540800381730, 1.000000000000000000 ) ) 
 REPRESENTATION_ITEM ( '' )  );
#22106=ORIENTED_EDGE ( 'NONE', *, *, #9724, .F. ) ;
#22140=ORIENTED_EDGE ( 'NONE', *, *, #21976, .T. ) ;
#22142=EDGE_LOOP ( 'NONE', ( #5245, #9832, #12107, #3534 ) ) ;
#22170=AXIS2_PLACEMENT_3D ( 'NONE', #20345, #11766, #7809 ) ;
#22181=DIRECTION ( 'NONE',  ( 0.7071067811864976127, 0.000000000000000000, -0.7071067811865975328 ) ) ;
#22210=DIRECTION ( 'NONE',  ( 0.000000000000000000, 1.000000000000000000, 0.000000000000000000 ) ) ;
#22211=VERTEX_POINT ( 'NONE', #21326 ) ;
#22223=ORIENTED_EDGE ( 'NONE', *, *, #7072, .T. ) ;
#22238=ORIENTED_EDGE ( 'NONE', *, *, #20236, .F. ) ;
#22248=AXIS2_PLACEMENT_3D ( 'NONE', #10935, #14694, #7535 ) ;
#22254=LINE ( 'NONE', #20394, #13698 ) ;
#22259=DIRECTION ( 'NONE',  ( -0.000000000000000000, 1.000000000000000000, 0.000000000000000000 ) ) ;
#22269=ORIENTED_EDGE ( 'NONE', *, *, #8235, .T. ) ;
#22272=DIRECTION ( 'NONE',  ( 0.000000000000000000, 0.000000000000000000, -1.000000000000000000 ) ) ;
#22302=CIRCLE ( 'NONE', #20442, 0.7620000000000366480 ) ;
#22307=SPHERICAL_SURFACE ( 'NONE', #3405, 0.7620000000000000107 ) ;
#22313=ORIENTED_EDGE ( 'NONE', *, *, #16655, .F. ) ;
#22334=ORIENTED_EDGE ( 'NONE', *, *, #8356, .T. ) ;
#22356=ORIENTED_EDGE ( 'NONE', *, *, #14571, .T. ) ;
#22365=VERTEX_POINT ( 'NONE', #18828 ) ;
#22369=CIRCLE ( 'NONE', #5561, 6.476999999999001112 ) ;
#22378=LINE ( 'NONE', #18873, #5158 ) ;
#22393=DIRECTION ( 'NONE',  ( -1.000000000000000000, 0.000000000000000000, 0.000000000000000000 ) ) ;
#22400=DIRECTION ( 'NONE',  ( 0.000000000000000000, -1.000000000000000000, 0.000000000000000000 ) ) ;
#22409=VERTEX_POINT ( 'NONE', #21064 ) ;
#22410=EDGE_LOOP ( 'NONE', ( #100, #9366, #10399, #18072 ) ) ;
#22420=AXIS2_PLACEMENT_3D ( 'NONE', #16786, #629, #20422 ) ;
#22421=DIRECTION ( 'NONE',  ( 0.7071067811865703323, 0.000000000000000000, 0.7071067811865248132 ) ) ;
#22441=EDGE_CURVE ( 'NONE', #20566, #14108, #22776, .T. ) ;
#22456=AXIS2_PLACEMENT_3D ( 'NONE', #17941, #21471, #17834 ) ;
#22461=EDGE_CURVE ( 'NONE', #18833, #5647, #1439, .T. ) ;
#22503=PLANE ( 'NONE',  #11043 ) ;
#22504=EDGE_CURVE ( 'NONE', #19328, #15238, #330, .T. ) ;
#22509=ORIENTED_EDGE ( 'NONE', *, *, #11516, .F. ) ;
#22514=EDGE_CURVE ( 'NONE', #7880, #11168, #13432, .T. ) ;
#22518=CARTESIAN_POINT ( 'NONE',  ( 20.32000000000000028, -3568.700000000000273, 2292.057900000000245 ) ) ;
#22531=FACE_OUTER_BOUND ( 'NONE', #10852, .T. ) ;
#22542=EDGE_CURVE ( 'NONE', #20662, #11168, #82, .T. ) ;
#22549=ADVANCED_FACE ( 'NONE', ( #8983 ), #11199, .T. ) ;
#22562=CIRCLE ( 'NONE', #19217, 0.7619999999999294005 ) ;
#22565=CIRCLE ( 'NONE', #504, 0.7620000000000000107 ) ;
#22571=DIRECTION ( 'NONE',  ( 0.000000000000000000, 0.000000000000000000, -1.000000000000000000 ) ) ;
#22616=CARTESIAN_POINT ( 'NONE',  ( 20.32000000000000028, -3544.061999999999898, 2292.057900000000245 ) ) ;
#22623=AXIS2_PLACEMENT_3D ( 'NONE', #12353, #20788, #10474 ) ;
#22624=ORIENTED_EDGE ( 'NONE', *, *, #9302, .F. ) ;
#22644=CIRCLE ( 'NONE', #9932, 0.7619999999999294005 ) ;
#22673=CIRCLE ( 'NONE', #18932, 2.844800000000091700 ) ;
#22676=DIRECTION ( 'NONE',  ( 1.000000000000000000, 0.000000000000000000, 0.000000000000000000 ) ) ;
#22706=FACE_OUTER_BOUND ( 'NONE', #14923, .T. ) ;
#22716=CARTESIAN_POINT ( 'NONE',  ( 20.32000000000000028, -3568.700000000000273, 2289.213099999999940 ) ) ;
#22727=ORIENTED_EDGE ( 'NONE', *, *, #21970, .T. ) ;
#22730=AXIS2_PLACEMENT_3D ( 'NONE', #208, #17656, #7359 ) ;
#22732=DIRECTION ( 'NONE',  ( 1.678948246106317188E-14, 0.000000000000000000, -1.000000000000000000 ) ) ;
#22767=VERTEX_POINT ( 'NONE', #14953 ) ;
#22768=ORIENTED_EDGE ( 'NONE', *, *, #12163, .F. ) ;
#22769=CARTESIAN_POINT ( 'NONE',  ( 20.32000000000000028, -3670.300000000000182, 2292.057900000000245 ) ) ;
#22776=CIRCLE ( 'NONE', #9674, 0.7619999999999294005 ) ;
#22789=AXIS2_PLACEMENT_3D ( 'NONE', #18232, #7915, #4167 ) ;
#22793=VERTEX_POINT ( 'NONE', #20453 ) ;
#22802=EDGE_CURVE ( 'NONE', #6791, #20799, #14951, .T. ) ;
#22804=DIRECTION ( 'NONE',  ( -1.000000000000000000, 0.000000000000000000, 0.000000000000000000 ) ) ;
#22811=EDGE_CURVE ( 'NONE', #19948, #17590, #19821, .T. ) ;
#22814=CARTESIAN_POINT ( 'NONE',  ( 12.69999999999999929, -3599.497499999999945, 2288.971800000000258 ) ) ;
#22817=EDGE_CURVE ( 'NONE', #1200, #18510, #2301, .T. ) ;
#22825=DIRECTION ( 'NONE',  ( 0.000000000000000000, 1.000000000000000000, 0.000000000000000000 ) ) ;
#22831=CARTESIAN_POINT ( 'NONE',  ( 22.54063073453000143, -3543.299999999999727, 2275.763800000000174 ) ) ;
#22874=EDGE_LOOP ( 'NONE', ( #18133, #392 ) ) ;
#22881=ORIENTED_EDGE ( 'NONE', *, *, #8516, .F. ) ;
#22890=DIRECTION ( 'NONE',  ( 0.000000000000000000, 0.000000000000000000, 1.000000000000000000 ) ) ;
#22892=VECTOR ( 'NONE', #9204, 1000.000000000000000 ) ;
#22895=ORIENTED_EDGE ( 'NONE', *, *, #14329, .T. ) ;
#22900=EDGE_CURVE ( 'NONE', #10742, #16618, #21314, .T. ) ;
#22914=CIRCLE ( 'NONE', #21812, 0.7620000000000000107 ) ;
#22935=DIRECTION ( 'NONE',  ( 0.7071067811865975328, 0.000000000000000000, -0.7071067811864976127 ) ) ;
#22963=DIRECTION ( 'NONE',  ( 0.000000000000000000, 0.000000000000000000, 1.000000000000000000 ) ) ;
#22996=EDGE_CURVE ( 'NONE', #17905, #20779, #2609, .T. ) ;
#23022=CARTESIAN_POINT ( 'NONE',  ( 61.26424768829000556, -3694.938000000000102, 2279.065800000000309 ) ) ;
#23029=ORIENTED_EDGE ( 'NONE', *, *, #15026, .T. ) ;
#23034=CIRCLE ( 'NONE', #12579, 0.7619999999999294005 ) ;
#23048=DIRECTION ( 'NONE',  ( 0.000000000000000000, -1.000000000000000000, 0.000000000000000000 ) ) ;
#23050=TOROIDAL_SURFACE ( 'NONE', #7731, 1.524000000000000021, 0.7620000000000000107 ) ;
#23051=ADVANCED_FACE ( 'NONE', ( #3563, #1927, #7321 ), #5573, .F. ) ;
#23072=DIRECTION ( 'NONE',  ( 0.000000000000000000, -1.000000000000000000, 0.000000000000000000 ) ) ;
#23084=DIRECTION ( 'NONE',  ( 0.000000000000000000, -1.000000000000000000, 0.000000000000000000 ) ) ;
#23092=CARTESIAN_POINT ( 'NONE',  ( 9.855199999999999960, -3599.497499999999945, 2281.351799999999912 ) ) ;
#23094=( NAMED_UNIT ( * ) SI_UNIT ( $, .STERADIAN. ) SOLID_ANGLE_UNIT ( ) );
#23110=AXIS2_PLACEMENT_3D ( 'NONE', #19782, #10865, #1845 ) ;
#23123=DIRECTION ( 'NONE',  ( 0.000000000000000000, 0.000000000000000000, -1.000000000000000000 ) ) ;
#23127=ORIENTED_EDGE ( 'NONE', *, *, #15959, .T. ) ;
#23150=ORIENTED_EDGE ( 'NONE', *, *, #20010, .F. ) ;
#23159=EDGE_CURVE ( 'NONE', #21628, #1371, #13845, .T. ) ;
#23187=COLOUR_RGB('Light Blue',0.38,0.62,0.78);
#23188=FILL_AREA_STYLE_COLOUR('',#23187);
#23189=FILL_AREA_STYLE('',(#23188));
#23190=SURFACE_STYLE_FILL_AREA(#23189);
#23191=SURFACE_SIDE_STYLE('',(#23190));
#23192=SURFACE_STYLE_USAGE(.BOTH.,#23191);
#23193=PRESENTATION_STYLE_ASSIGNMENT((#23192));
#23231=STYLED_ITEM('',(#23193),#13285);
#23237=MECHANICAL_DESIGN_GEOMETRIC_PRESENTATION_REPRESENTATION('',(#23231),#2257);
ENDSEC;
END-ISO-10303-21;
